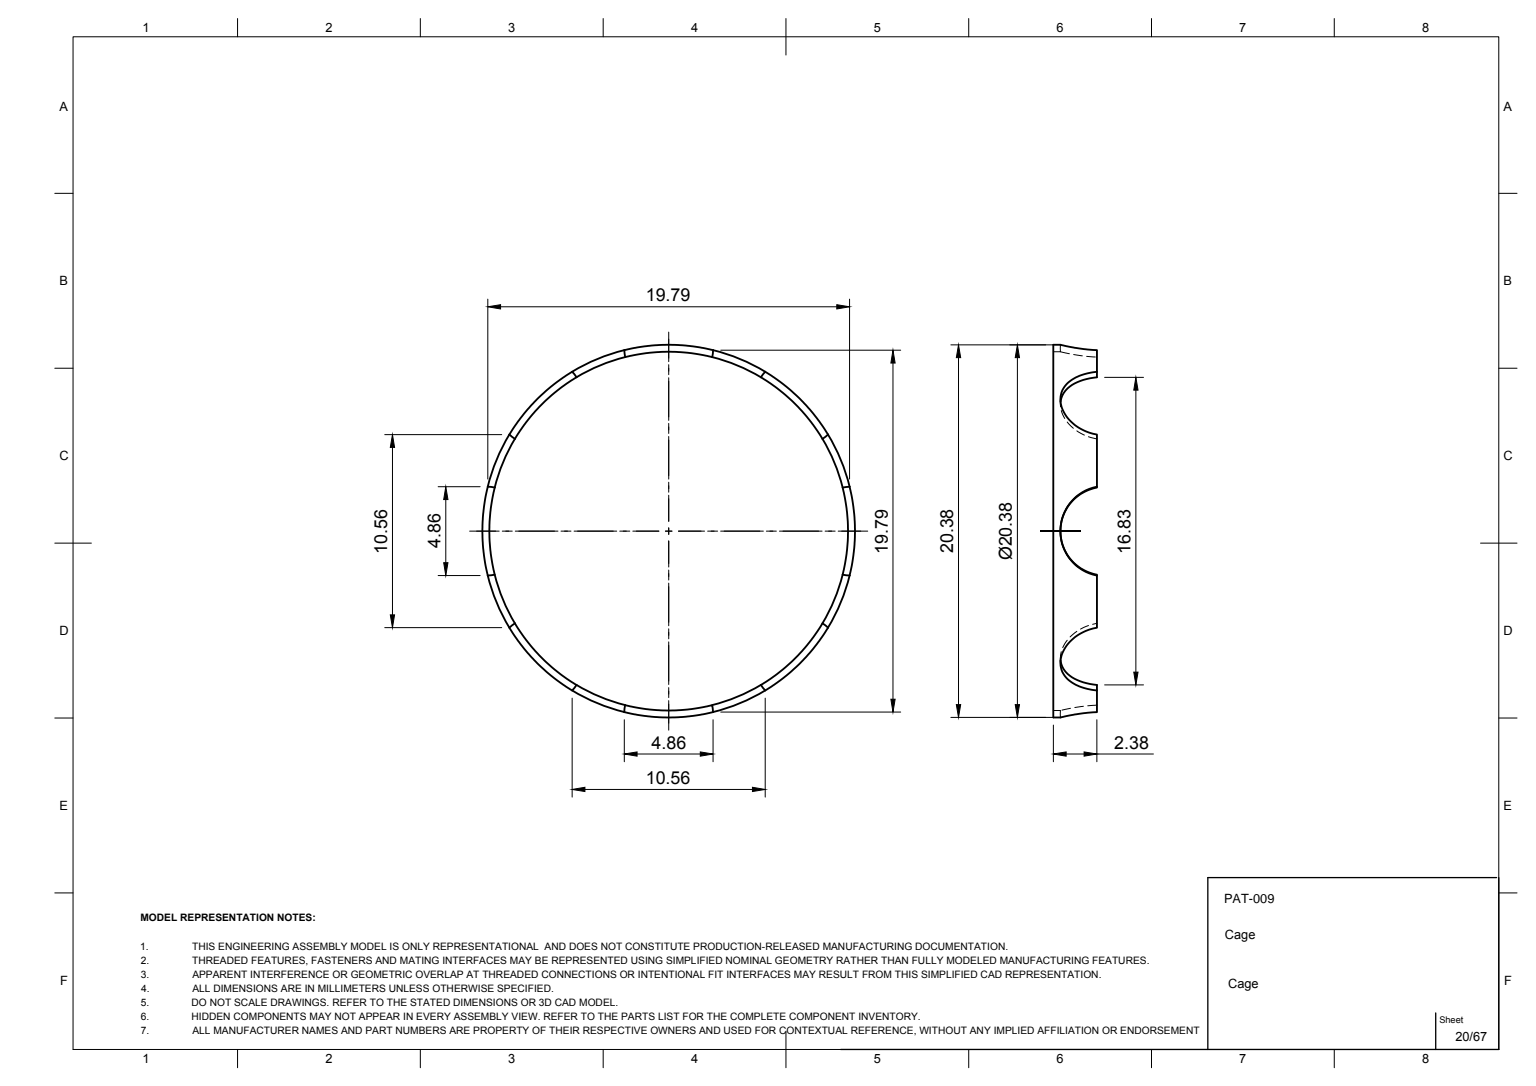
ISO-10303-21;
HEADER;
/* Generated by software containing ST-Developer
 * from STEP Tools, Inc. (www.steptools.com) 
 */

FILE_DESCRIPTION(
/* description */ ('Bell-crank linkage with push rods'),
/* implementation_level */ '2;1');

FILE_NAME(
/* name */ 'Cage.step',
/* time_stamp */ '2026-10-28T03:25:15-07:00',
/* author */ (''),
/* organization */ (''),
/* preprocessor_version */ 'ST-DEVELOPER v20.2',
/* originating_system */ 'Autodesk Translation Framework v15.17.0.0',
/* authorisation */ '');

FILE_SCHEMA (('AUTOMOTIVE_DESIGN { 1 0 10303 214 3 1 1 }'));
ENDSEC;

DATA;
#10=MECHANICAL_DESIGN_GEOMETRIC_PRESENTATION_REPRESENTATION('',(#624),#16678);
#423=SPHERICAL_SURFACE('',#9847,0.247676);
#424=SPHERICAL_SURFACE('',#9863,0.247676);
#425=SPHERICAL_SURFACE('',#9868,0.247676);
#426=SPHERICAL_SURFACE('',#9873,0.247676);
#427=SPHERICAL_SURFACE('',#9878,0.247676);
#428=SPHERICAL_SURFACE('',#9883,0.247676);
#429=SPHERICAL_SURFACE('',#9888,0.247676);
#430=SPHERICAL_SURFACE('',#9896,0.247676);
#473=B_SPLINE_CURVE_WITH_KNOTS('',3,(#14583,#14584,#14585,#14586,#14587,
#14588,#14589,#14590,#14591,#14592,#14593,#14594,#14595,#14596,#14597,#14598,
#14599,#14600,#14601,#14602,#14603,#14604),.UNSPECIFIED.,.F.,.F.,(4,2,2,
2,2,2,2,2,2,2,4),(0.0473477652366656,0.126350602536658,0.189525903804987,
0.252701205073317,0.313298422430275,0.373895639787233,0.434492857144191,
0.495090074501149,0.558265375769478,0.621440677037807,0.7004435143378),
 .UNSPECIFIED.);
#474=B_SPLINE_CURVE_WITH_KNOTS('',3,(#14608,#14609,#14610,#14611,#14612,
#14613,#14614,#14615,#14616,#14617,#14618,#14619,#14620,#14621,#14622,#14623,
#14624,#14625,#14626,#14627,#14628,#14629),.UNSPECIFIED.,.F.,.F.,(4,2,2,
2,2,2,2,2,2,2,4),(0.0464897534940957,0.0852567806515119,0.170513561303024,
0.246687263103517,0.308657850341199,0.370628437578881,0.432599024816563,
0.494569612054245,0.570743313854739,0.656000094506251,0.694767121663666),
 .UNSPECIFIED.);
#475=B_SPLINE_CURVE_WITH_KNOTS('',3,(#14635,#14636,#14637,#14638,#14639,
#14640,#14641,#14642,#14643,#14644,#14645,#14646,#14647,#14648,#14649,#14650,
#14651,#14652,#14653,#14654,#14655,#14656),.UNSPECIFIED.,.F.,.F.,(4,2,2,
2,2,2,2,2,2,2,4),(0.0464897534940957,0.0852567806515118,0.170513561303024,
0.246687263103517,0.308657850341199,0.370628437578881,0.432599024816563,
0.494569612054245,0.570743313854738,0.65600009450625,0.694767121663666),
 .UNSPECIFIED.);
#476=B_SPLINE_CURVE_WITH_KNOTS('',3,(#14660,#14661,#14662,#14663,#14664,
#14665,#14666,#14667,#14668,#14669,#14670,#14671,#14672,#14673,#14674,#14675,
#14676,#14677,#14678,#14679,#14680,#14681),.UNSPECIFIED.,.F.,.F.,(4,2,2,
2,2,2,2,2,2,2,4),(0.0464897534940957,0.0852567806515119,0.170513561303024,
0.246687263103517,0.308657850341199,0.370628437578881,0.432599024816563,
0.494569612054245,0.570743313854739,0.656000094506251,0.694767121663666),
 .UNSPECIFIED.);
#477=B_SPLINE_CURVE_WITH_KNOTS('',3,(#14685,#14686,#14687,#14688,#14689,
#14690,#14691,#14692,#14693,#14694,#14695,#14696),.UNSPECIFIED.,.F.,.F.,
(4,2,2,2,2,4),(0.0464897534940957,0.0852567806515119,0.170513561303024,
0.246687263103517,0.308657850341199,0.370628437578881),.UNSPECIFIED.);
#478=B_SPLINE_CURVE_WITH_KNOTS('',3,(#14701,#14702,#14703,#14704,#14705,
#14706,#14707,#14708,#14709,#14710,#14711,#14712),.UNSPECIFIED.,.F.,.F.,
(4,2,2,2,2,4),(0.370628437578881,0.432599024816563,0.494569612054245,0.570743313854738,
0.65600009450625,0.694767121663666),.UNSPECIFIED.);
#479=B_SPLINE_CURVE_WITH_KNOTS('',3,(#14716,#14717,#14718,#14719,#14720,
#14721,#14722,#14723,#14724,#14725,#14726,#14727,#14728,#14729,#14730,#14731,
#14732,#14733,#14734,#14735,#14736,#14737),.UNSPECIFIED.,.F.,.F.,(4,2,2,
2,2,2,2,2,2,2,4),(0.0464897534940957,0.0852567806515121,0.170513561303024,
0.246687263103518,0.308657850341199,0.370628437578881,0.432599024816563,
0.494569612054245,0.570743313854738,0.65600009450625,0.694767121663666),
 .UNSPECIFIED.);
#480=B_SPLINE_CURVE_WITH_KNOTS('',3,(#14741,#14742,#14743,#14744,#14745,
#14746,#14747,#14748,#14749,#14750,#14751,#14752,#14753,#14754,#14755,#14756,
#14757,#14758,#14759,#14760,#14761,#14762),.UNSPECIFIED.,.F.,.F.,(4,2,2,
2,2,2,2,2,2,2,4),(0.0464897534940957,0.0852567806515119,0.170513561303024,
0.246687263103517,0.308657850341199,0.370628437578881,0.432599024816563,
0.494569612054245,0.570743313854738,0.65600009450625,0.694767121663667),
 .UNSPECIFIED.);
#481=B_SPLINE_CURVE_WITH_KNOTS('',3,(#14766,#14767,#14768,#14769,#14770,
#14771,#14772,#14773,#14774,#14775,#14776,#14777,#14778,#14779,#14780,#14781,
#14782,#14783,#14784,#14785,#14786,#14787),.UNSPECIFIED.,.F.,.F.,(4,2,2,
2,2,2,2,2,2,2,4),(0.0464897534940957,0.0852567806515119,0.170513561303024,
0.246687263103517,0.308657850341199,0.370628437578881,0.432599024816563,
0.494569612054245,0.570743313854738,0.65600009450625,0.694767121663666),
 .UNSPECIFIED.);
#482=B_SPLINE_CURVE_WITH_KNOTS('',3,(#14791,#14792,#14793,#14794,#14795,
#14796,#14797,#14798,#14799,#14800,#14801,#14802,#14803,#14804,#14805,#14806,
#14807,#14808,#14809,#14810,#14811,#14812),.UNSPECIFIED.,.F.,.F.,(4,2,2,
2,2,2,2,2,2,2,4),(0.0464897534940957,0.0852567806515119,0.170513561303024,
0.246687263103517,0.308657850341199,0.370628437578881,0.432599024816563,
0.494569612054245,0.570743313854739,0.656000094506251,0.694767121663667),
 .UNSPECIFIED.);
#483=B_SPLINE_CURVE_WITH_KNOTS('',3,(#14820,#14821,#14822,#14823,#14824,
#14825,#14826,#14827,#14828,#14829,#14830,#14831,#14832,#14833,#14834,#14835,
#14836,#14837,#14838,#14839,#14840,#14841),.UNSPECIFIED.,.F.,.F.,(4,2,2,
2,2,2,2,2,2,2,4),(0.0473477652366656,0.126350602536658,0.189525903804987,
0.252701205073316,0.313298422430274,0.373895639787232,0.434492857144191,
0.495090074501149,0.558265375769478,0.621440677037807,0.7004435143378),
 .UNSPECIFIED.);
#484=B_SPLINE_CURVE_WITH_KNOTS('',3,(#14849,#14850,#14851,#14852,#14853,
#14854,#14855,#14856,#14857,#14858,#14859,#14860,#14861,#14862,#14863,#14864,
#14865,#14866,#14867,#14868,#14869,#14870),.UNSPECIFIED.,.F.,.F.,(4,2,2,
2,2,2,2,2,2,2,4),(0.0473477652366656,0.126350602536658,0.189525903804987,
0.252701205073317,0.313298422430275,0.373895639787233,0.434492857144191,
0.495090074501149,0.558265375769478,0.621440677037807,0.7004435143378),
 .UNSPECIFIED.);
#485=B_SPLINE_CURVE_WITH_KNOTS('',3,(#14879,#14880,#14881,#14882,#14883,
#14884,#14885,#14886,#14887,#14888,#14889,#14890),.UNSPECIFIED.,.F.,.F.,
(4,2,2,2,2,4),(0.0473477652366656,0.126350602536658,0.189525903804987,0.252701205073316,
0.313298422430275,0.373895639787233),.UNSPECIFIED.);
#486=B_SPLINE_CURVE_WITH_KNOTS('',3,(#14892,#14893,#14894,#14895,#14896,
#14897,#14898,#14899,#14900,#14901,#14902,#14903),.UNSPECIFIED.,.F.,.F.,
(4,2,2,2,2,4),(0.373895639787233,0.434492857144191,0.495090074501149,0.558265375769478,
0.621440677037807,0.7004435143378),.UNSPECIFIED.);
#487=B_SPLINE_CURVE_WITH_KNOTS('',3,(#14910,#14911,#14912,#14913,#14914,
#14915,#14916,#14917,#14918,#14919,#14920,#14921,#14922,#14923,#14924,#14925,
#14926,#14927,#14928,#14929,#14930,#14931),.UNSPECIFIED.,.F.,.F.,(4,2,2,
2,2,2,2,2,2,2,4),(0.0473477652366656,0.126350602536658,0.189525903804987,
0.252701205073316,0.313298422430275,0.373895639787233,0.434492857144191,
0.495090074501149,0.558265375769478,0.621440677037807,0.7004435143378),
 .UNSPECIFIED.);
#488=B_SPLINE_CURVE_WITH_KNOTS('',3,(#14939,#14940,#14941,#14942,#14943,
#14944,#14945,#14946,#14947,#14948,#14949,#14950,#14951,#14952,#14953,#14954,
#14955,#14956,#14957,#14958,#14959,#14960),.UNSPECIFIED.,.F.,.F.,(4,2,2,
2,2,2,2,2,2,2,4),(0.0473477652366656,0.126350602536658,0.189525903804987,
0.252701205073317,0.313298422430275,0.373895639787233,0.434492857144191,
0.495090074501149,0.558265375769478,0.621440677037807,0.7004435143378),
 .UNSPECIFIED.);
#489=B_SPLINE_CURVE_WITH_KNOTS('',3,(#14968,#14969,#14970,#14971,#14972,
#14973,#14974,#14975,#14976,#14977,#14978,#14979,#14980,#14981,#14982,#14983,
#14984,#14985,#14986,#14987,#14988,#14989),.UNSPECIFIED.,.F.,.F.,(4,2,2,
2,2,2,2,2,2,2,4),(0.0473477652366656,0.126350602536658,0.189525903804987,
0.252701205073316,0.313298422430275,0.373895639787233,0.434492857144191,
0.495090074501149,0.558265375769478,0.621440677037807,0.7004435143378),
 .UNSPECIFIED.);
#490=B_SPLINE_CURVE_WITH_KNOTS('',3,(#14998,#14999,#15000,#15001,#15002,
#15003,#15004,#15005,#15006,#15007,#15008,#15009,#15010,#15011,#15012,#15013,
#15014,#15015,#15016,#15017,#15018,#15019),.UNSPECIFIED.,.F.,.F.,(4,2,2,
2,2,2,2,2,2,2,4),(0.0473477652366656,0.126350602536658,0.189525903804987,
0.252701205073317,0.313298422430275,0.373895639787233,0.434492857144191,
0.495090074501149,0.558265375769478,0.621440677037807,0.7004435143378),
 .UNSPECIFIED.);
#509=SHAPE_REPRESENTATION_RELATIONSHIP('SRR','None',#16926,#563);
#563=ADVANCED_BREP_SHAPE_REPRESENTATION('',(#685),#16631);
#624=STYLED_ITEM('',(#17291),#685);
#685=MANIFOLD_SOLID_BREP('Continuous crown cage',#8815);
#817=FACE_BOUND('',#2066,.T.);
#1058=PLANE('',#9860);
#1059=PLANE('',#9865);
#1060=PLANE('',#9870);
#1061=PLANE('',#9875);
#1062=PLANE('',#9880);
#1063=PLANE('',#9885);
#1064=PLANE('',#9894);
#1065=PLANE('',#9898);
#1066=PLANE('',#9899);
#1434=FACE_OUTER_BOUND('',#2048,.T.);
#1435=FACE_OUTER_BOUND('',#2049,.T.);
#1436=FACE_OUTER_BOUND('',#2050,.T.);
#1437=FACE_OUTER_BOUND('',#2051,.T.);
#1438=FACE_OUTER_BOUND('',#2052,.T.);
#1439=FACE_OUTER_BOUND('',#2053,.T.);
#1440=FACE_OUTER_BOUND('',#2054,.T.);
#1441=FACE_OUTER_BOUND('',#2055,.T.);
#1442=FACE_OUTER_BOUND('',#2056,.T.);
#1443=FACE_OUTER_BOUND('',#2057,.T.);
#1444=FACE_OUTER_BOUND('',#2058,.T.);
#1445=FACE_OUTER_BOUND('',#2059,.T.);
#1446=FACE_OUTER_BOUND('',#2060,.T.);
#1447=FACE_OUTER_BOUND('',#2061,.T.);
#1448=FACE_OUTER_BOUND('',#2062,.T.);
#1449=FACE_OUTER_BOUND('',#2063,.T.);
#1450=FACE_OUTER_BOUND('',#2064,.T.);
#1451=FACE_OUTER_BOUND('',#2065,.T.);
#1452=FACE_OUTER_BOUND('',#2067,.T.);
#2048=EDGE_LOOP('',(#6755,#6756,#6757,#6758));
#2049=EDGE_LOOP('',(#6759,#6760,#6761,#6762,#6763,#6764,#6765,#6766,#6767,
#6768,#6769,#6770,#6771,#6772,#6773,#6774,#6775,#6776,#6777,#6778));
#2050=EDGE_LOOP('',(#6779,#6780,#6781,#6782));
#2051=EDGE_LOOP('',(#6783,#6784,#6785,#6786));
#2052=EDGE_LOOP('',(#6787,#6788,#6789,#6790));
#2053=EDGE_LOOP('',(#6791,#6792,#6793,#6794));
#2054=EDGE_LOOP('',(#6795,#6796,#6797,#6798));
#2055=EDGE_LOOP('',(#6799,#6800,#6801,#6802,#6803,#6804));
#2056=EDGE_LOOP('',(#6805,#6806,#6807,#6808));
#2057=EDGE_LOOP('',(#6809,#6810,#6811,#6812));
#2058=EDGE_LOOP('',(#6813,#6814,#6815,#6816));
#2059=EDGE_LOOP('',(#6817,#6818,#6819,#6820));
#2060=EDGE_LOOP('',(#6821,#6822,#6823,#6824));
#2061=EDGE_LOOP('',(#6825,#6826,#6827,#6828));
#2062=EDGE_LOOP('',(#6829,#6830,#6831,#6832,#6833,#6834,#6835,#6836,#6837,
#6838,#6839,#6840,#6841,#6842,#6843,#6844,#6845,#6846,#6847,#6848));
#2063=EDGE_LOOP('',(#6849,#6850,#6851,#6852));
#2064=EDGE_LOOP('',(#6853,#6854,#6855,#6856));
#2065=EDGE_LOOP('',(#6857));
#2066=EDGE_LOOP('',(#6858));
#2067=EDGE_LOOP('',(#6859,#6860,#6861,#6862));
#2749=LINE('',#14698,#3298);
#2750=LINE('',#14994,#3299);
#3298=VECTOR('',#11647,1.019052);
#3299=VECTOR('',#11724,0.980948);
#3819=CIRCLE('',#9848,0.243053047864041);
#3820=CIRCLE('',#9849,0.243053047864041);
#3821=CIRCLE('',#9851,1.019052);
#3822=CIRCLE('',#9852,1.019052);
#3823=CIRCLE('',#9853,1.019052);
#3824=CIRCLE('',#9854,1.019052);
#3825=CIRCLE('',#9855,1.019052);
#3826=CIRCLE('',#9856,1.019052);
#3827=CIRCLE('',#9857,1.019052);
#3828=CIRCLE('',#9858,1.019052);
#3829=CIRCLE('',#9859,1.019052);
#3830=CIRCLE('',#9861,0.980948);
#3831=CIRCLE('',#9862,0.243053047864041);
#3832=CIRCLE('',#9864,0.243053047864041);
#3833=CIRCLE('',#9866,0.980948);
#3834=CIRCLE('',#9867,0.243053047864041);
#3835=CIRCLE('',#9869,0.243053047864041);
#3836=CIRCLE('',#9871,0.980948);
#3837=CIRCLE('',#9872,0.243053047864041);
#3838=CIRCLE('',#9874,0.243053047864041);
#3839=CIRCLE('',#9876,0.980948);
#3840=CIRCLE('',#9877,0.243053047864041);
#3841=CIRCLE('',#9879,0.243053047864041);
#3842=CIRCLE('',#9881,0.980948);
#3843=CIRCLE('',#9882,0.243053047864041);
#3844=CIRCLE('',#9884,0.243053047864041);
#3845=CIRCLE('',#9886,0.980948);
#3846=CIRCLE('',#9887,0.243053047864041);
#3847=CIRCLE('',#9889,0.243053047864041);
#3848=CIRCLE('',#9891,0.980948);
#3849=CIRCLE('',#9892,0.980948);
#3850=CIRCLE('',#9893,0.980948);
#3851=CIRCLE('',#9895,0.243053047864041);
#3852=CIRCLE('',#9897,0.243053047864041);
#4399=VERTEX_POINT('',#14581);
#4400=VERTEX_POINT('',#14582);
#4401=VERTEX_POINT('',#14605);
#4402=VERTEX_POINT('',#14607);
#4403=VERTEX_POINT('',#14632);
#4404=VERTEX_POINT('',#14634);
#4405=VERTEX_POINT('',#14657);
#4406=VERTEX_POINT('',#14659);
#4407=VERTEX_POINT('',#14682);
#4408=VERTEX_POINT('',#14684);
#4409=VERTEX_POINT('',#14697);
#4410=VERTEX_POINT('',#14700);
#4411=VERTEX_POINT('',#14713);
#4412=VERTEX_POINT('',#14715);
#4413=VERTEX_POINT('',#14738);
#4414=VERTEX_POINT('',#14740);
#4415=VERTEX_POINT('',#14763);
#4416=VERTEX_POINT('',#14765);
#4417=VERTEX_POINT('',#14788);
#4418=VERTEX_POINT('',#14790);
#4419=VERTEX_POINT('',#14815);
#4420=VERTEX_POINT('',#14819);
#4421=VERTEX_POINT('',#14844);
#4422=VERTEX_POINT('',#14848);
#4423=VERTEX_POINT('',#14873);
#4424=VERTEX_POINT('',#14877);
#4425=VERTEX_POINT('',#14878);
#4426=VERTEX_POINT('',#14905);
#4427=VERTEX_POINT('',#14909);
#4428=VERTEX_POINT('',#14934);
#4429=VERTEX_POINT('',#14938);
#4430=VERTEX_POINT('',#14963);
#4431=VERTEX_POINT('',#14967);
#4432=VERTEX_POINT('',#14992);
#4433=VERTEX_POINT('',#14995);
#4434=VERTEX_POINT('',#14997);
#5255=EDGE_CURVE('',#4399,#4400,#473,.T.);
#5256=EDGE_CURVE('',#4401,#4399,#3819,.T.);
#5257=EDGE_CURVE('',#4402,#4401,#474,.T.);
#5258=EDGE_CURVE('',#4400,#4402,#3820,.T.);
#5259=EDGE_CURVE('',#4403,#4401,#3821,.T.);
#5260=EDGE_CURVE('',#4403,#4404,#475,.T.);
#5261=EDGE_CURVE('',#4405,#4404,#3822,.T.);
#5262=EDGE_CURVE('',#4405,#4406,#476,.T.);
#5263=EDGE_CURVE('',#4407,#4406,#3823,.T.);
#5264=EDGE_CURVE('',#4407,#4408,#477,.T.);
#5265=EDGE_CURVE('',#4408,#4409,#2749,.T.);
#5266=EDGE_CURVE('',#4409,#4409,#3824,.T.);
#5267=EDGE_CURVE('',#4408,#4410,#478,.T.);
#5268=EDGE_CURVE('',#4411,#4410,#3825,.T.);
#5269=EDGE_CURVE('',#4411,#4412,#479,.T.);
#5270=EDGE_CURVE('',#4413,#4412,#3826,.T.);
#5271=EDGE_CURVE('',#4413,#4414,#480,.T.);
#5272=EDGE_CURVE('',#4415,#4414,#3827,.T.);
#5273=EDGE_CURVE('',#4415,#4416,#481,.T.);
#5274=EDGE_CURVE('',#4417,#4416,#3828,.T.);
#5275=EDGE_CURVE('',#4417,#4418,#482,.T.);
#5276=EDGE_CURVE('',#4402,#4418,#3829,.T.);
#5277=EDGE_CURVE('',#4399,#4419,#3830,.T.);
#5278=EDGE_CURVE('',#4419,#4403,#3831,.T.);
#5279=EDGE_CURVE('',#4420,#4419,#483,.T.);
#5280=EDGE_CURVE('',#4404,#4420,#3832,.T.);
#5281=EDGE_CURVE('',#4420,#4421,#3833,.T.);
#5282=EDGE_CURVE('',#4421,#4405,#3834,.T.);
#5283=EDGE_CURVE('',#4422,#4421,#484,.T.);
#5284=EDGE_CURVE('',#4406,#4422,#3835,.T.);
#5285=EDGE_CURVE('',#4422,#4423,#3836,.T.);
#5286=EDGE_CURVE('',#4423,#4407,#3837,.T.);
#5287=EDGE_CURVE('',#4424,#4425,#485,.T.);
#5288=EDGE_CURVE('',#4410,#4424,#3838,.T.);
#5289=EDGE_CURVE('',#4425,#4423,#486,.T.);
#5290=EDGE_CURVE('',#4424,#4426,#3839,.T.);
#5291=EDGE_CURVE('',#4426,#4411,#3840,.T.);
#5292=EDGE_CURVE('',#4427,#4426,#487,.T.);
#5293=EDGE_CURVE('',#4412,#4427,#3841,.T.);
#5294=EDGE_CURVE('',#4427,#4428,#3842,.T.);
#5295=EDGE_CURVE('',#4428,#4413,#3843,.T.);
#5296=EDGE_CURVE('',#4429,#4428,#488,.T.);
#5297=EDGE_CURVE('',#4414,#4429,#3844,.T.);
#5298=EDGE_CURVE('',#4429,#4430,#3845,.T.);
#5299=EDGE_CURVE('',#4430,#4415,#3846,.T.);
#5300=EDGE_CURVE('',#4431,#4430,#489,.T.);
#5301=EDGE_CURVE('',#4416,#4431,#3847,.T.);
#5302=EDGE_CURVE('',#4432,#4432,#3848,.T.);
#5303=EDGE_CURVE('',#4432,#4425,#2750,.T.);
#5304=EDGE_CURVE('',#4433,#4400,#3849,.T.);
#5305=EDGE_CURVE('',#4433,#4434,#490,.T.);
#5306=EDGE_CURVE('',#4431,#4434,#3850,.T.);
#5307=EDGE_CURVE('',#4418,#4433,#3851,.T.);
#5308=EDGE_CURVE('',#4434,#4417,#3852,.T.);
#6755=ORIENTED_EDGE('',*,*,#5255,.F.);
#6756=ORIENTED_EDGE('',*,*,#5256,.F.);
#6757=ORIENTED_EDGE('',*,*,#5257,.F.);
#6758=ORIENTED_EDGE('',*,*,#5258,.F.);
#6759=ORIENTED_EDGE('',*,*,#5257,.T.);
#6760=ORIENTED_EDGE('',*,*,#5259,.F.);
#6761=ORIENTED_EDGE('',*,*,#5260,.T.);
#6762=ORIENTED_EDGE('',*,*,#5261,.F.);
#6763=ORIENTED_EDGE('',*,*,#5262,.T.);
#6764=ORIENTED_EDGE('',*,*,#5263,.F.);
#6765=ORIENTED_EDGE('',*,*,#5264,.T.);
#6766=ORIENTED_EDGE('',*,*,#5265,.T.);
#6767=ORIENTED_EDGE('',*,*,#5266,.F.);
#6768=ORIENTED_EDGE('',*,*,#5265,.F.);
#6769=ORIENTED_EDGE('',*,*,#5267,.T.);
#6770=ORIENTED_EDGE('',*,*,#5268,.F.);
#6771=ORIENTED_EDGE('',*,*,#5269,.T.);
#6772=ORIENTED_EDGE('',*,*,#5270,.F.);
#6773=ORIENTED_EDGE('',*,*,#5271,.T.);
#6774=ORIENTED_EDGE('',*,*,#5272,.F.);
#6775=ORIENTED_EDGE('',*,*,#5273,.T.);
#6776=ORIENTED_EDGE('',*,*,#5274,.F.);
#6777=ORIENTED_EDGE('',*,*,#5275,.T.);
#6778=ORIENTED_EDGE('',*,*,#5276,.F.);
#6779=ORIENTED_EDGE('',*,*,#5256,.T.);
#6780=ORIENTED_EDGE('',*,*,#5277,.T.);
#6781=ORIENTED_EDGE('',*,*,#5278,.T.);
#6782=ORIENTED_EDGE('',*,*,#5259,.T.);
#6783=ORIENTED_EDGE('',*,*,#5279,.F.);
#6784=ORIENTED_EDGE('',*,*,#5280,.F.);
#6785=ORIENTED_EDGE('',*,*,#5260,.F.);
#6786=ORIENTED_EDGE('',*,*,#5278,.F.);
#6787=ORIENTED_EDGE('',*,*,#5280,.T.);
#6788=ORIENTED_EDGE('',*,*,#5281,.T.);
#6789=ORIENTED_EDGE('',*,*,#5282,.T.);
#6790=ORIENTED_EDGE('',*,*,#5261,.T.);
#6791=ORIENTED_EDGE('',*,*,#5283,.F.);
#6792=ORIENTED_EDGE('',*,*,#5284,.F.);
#6793=ORIENTED_EDGE('',*,*,#5262,.F.);
#6794=ORIENTED_EDGE('',*,*,#5282,.F.);
#6795=ORIENTED_EDGE('',*,*,#5284,.T.);
#6796=ORIENTED_EDGE('',*,*,#5285,.T.);
#6797=ORIENTED_EDGE('',*,*,#5286,.T.);
#6798=ORIENTED_EDGE('',*,*,#5263,.T.);
#6799=ORIENTED_EDGE('',*,*,#5287,.F.);
#6800=ORIENTED_EDGE('',*,*,#5288,.F.);
#6801=ORIENTED_EDGE('',*,*,#5267,.F.);
#6802=ORIENTED_EDGE('',*,*,#5264,.F.);
#6803=ORIENTED_EDGE('',*,*,#5286,.F.);
#6804=ORIENTED_EDGE('',*,*,#5289,.F.);
#6805=ORIENTED_EDGE('',*,*,#5288,.T.);
#6806=ORIENTED_EDGE('',*,*,#5290,.T.);
#6807=ORIENTED_EDGE('',*,*,#5291,.T.);
#6808=ORIENTED_EDGE('',*,*,#5268,.T.);
#6809=ORIENTED_EDGE('',*,*,#5292,.F.);
#6810=ORIENTED_EDGE('',*,*,#5293,.F.);
#6811=ORIENTED_EDGE('',*,*,#5269,.F.);
#6812=ORIENTED_EDGE('',*,*,#5291,.F.);
#6813=ORIENTED_EDGE('',*,*,#5293,.T.);
#6814=ORIENTED_EDGE('',*,*,#5294,.T.);
#6815=ORIENTED_EDGE('',*,*,#5295,.T.);
#6816=ORIENTED_EDGE('',*,*,#5270,.T.);
#6817=ORIENTED_EDGE('',*,*,#5296,.F.);
#6818=ORIENTED_EDGE('',*,*,#5297,.F.);
#6819=ORIENTED_EDGE('',*,*,#5271,.F.);
#6820=ORIENTED_EDGE('',*,*,#5295,.F.);
#6821=ORIENTED_EDGE('',*,*,#5297,.T.);
#6822=ORIENTED_EDGE('',*,*,#5298,.T.);
#6823=ORIENTED_EDGE('',*,*,#5299,.T.);
#6824=ORIENTED_EDGE('',*,*,#5272,.T.);
#6825=ORIENTED_EDGE('',*,*,#5273,.F.);
#6826=ORIENTED_EDGE('',*,*,#5299,.F.);
#6827=ORIENTED_EDGE('',*,*,#5300,.F.);
#6828=ORIENTED_EDGE('',*,*,#5301,.F.);
#6829=ORIENTED_EDGE('',*,*,#5302,.F.);
#6830=ORIENTED_EDGE('',*,*,#5303,.T.);
#6831=ORIENTED_EDGE('',*,*,#5289,.T.);
#6832=ORIENTED_EDGE('',*,*,#5285,.F.);
#6833=ORIENTED_EDGE('',*,*,#5283,.T.);
#6834=ORIENTED_EDGE('',*,*,#5281,.F.);
#6835=ORIENTED_EDGE('',*,*,#5279,.T.);
#6836=ORIENTED_EDGE('',*,*,#5277,.F.);
#6837=ORIENTED_EDGE('',*,*,#5255,.T.);
#6838=ORIENTED_EDGE('',*,*,#5304,.F.);
#6839=ORIENTED_EDGE('',*,*,#5305,.T.);
#6840=ORIENTED_EDGE('',*,*,#5306,.F.);
#6841=ORIENTED_EDGE('',*,*,#5300,.T.);
#6842=ORIENTED_EDGE('',*,*,#5298,.F.);
#6843=ORIENTED_EDGE('',*,*,#5296,.T.);
#6844=ORIENTED_EDGE('',*,*,#5294,.F.);
#6845=ORIENTED_EDGE('',*,*,#5292,.T.);
#6846=ORIENTED_EDGE('',*,*,#5290,.F.);
#6847=ORIENTED_EDGE('',*,*,#5287,.T.);
#6848=ORIENTED_EDGE('',*,*,#5303,.F.);
#6849=ORIENTED_EDGE('',*,*,#5258,.T.);
#6850=ORIENTED_EDGE('',*,*,#5276,.T.);
#6851=ORIENTED_EDGE('',*,*,#5307,.T.);
#6852=ORIENTED_EDGE('',*,*,#5304,.T.);
#6853=ORIENTED_EDGE('',*,*,#5275,.F.);
#6854=ORIENTED_EDGE('',*,*,#5308,.F.);
#6855=ORIENTED_EDGE('',*,*,#5305,.F.);
#6856=ORIENTED_EDGE('',*,*,#5307,.F.);
#6857=ORIENTED_EDGE('',*,*,#5266,.T.);
#6858=ORIENTED_EDGE('',*,*,#5302,.T.);
#6859=ORIENTED_EDGE('',*,*,#5301,.T.);
#6860=ORIENTED_EDGE('',*,*,#5306,.T.);
#6861=ORIENTED_EDGE('',*,*,#5308,.T.);
#6862=ORIENTED_EDGE('',*,*,#5274,.T.);
#8145=CYLINDRICAL_SURFACE('',#9850,1.019052);
#8146=CYLINDRICAL_SURFACE('',#9890,0.980948);
#8459=ADVANCED_FACE('',(#1434),#423,.F.);
#8460=ADVANCED_FACE('',(#1435),#8145,.T.);
#8461=ADVANCED_FACE('',(#1436),#1058,.T.);
#8462=ADVANCED_FACE('',(#1437),#424,.F.);
#8463=ADVANCED_FACE('',(#1438),#1059,.T.);
#8464=ADVANCED_FACE('',(#1439),#425,.F.);
#8465=ADVANCED_FACE('',(#1440),#1060,.T.);
#8466=ADVANCED_FACE('',(#1441),#426,.F.);
#8467=ADVANCED_FACE('',(#1442),#1061,.T.);
#8468=ADVANCED_FACE('',(#1443),#427,.F.);
#8469=ADVANCED_FACE('',(#1444),#1062,.T.);
#8470=ADVANCED_FACE('',(#1445),#428,.F.);
#8471=ADVANCED_FACE('',(#1446),#1063,.T.);
#8472=ADVANCED_FACE('',(#1447),#429,.F.);
#8473=ADVANCED_FACE('',(#1448),#8146,.F.);
#8474=ADVANCED_FACE('',(#1449),#1064,.T.);
#8475=ADVANCED_FACE('',(#1450),#430,.F.);
#8476=ADVANCED_FACE('',(#1451,#817),#1065,.T.);
#8477=ADVANCED_FACE('',(#1452),#1066,.T.);
#8815=CLOSED_SHELL('',(#8459,#8460,#8461,#8462,#8463,#8464,#8465,#8466,
#8467,#8468,#8469,#8470,#8471,#8472,#8473,#8474,#8475,#8476,#8477));
#9846=AXIS2_PLACEMENT_3D('',#14579,#11631,#11632);
#9847=AXIS2_PLACEMENT_3D('',#14580,#11633,#11634);
#9848=AXIS2_PLACEMENT_3D('',#14606,#11635,#11636);
#9849=AXIS2_PLACEMENT_3D('',#14630,#11637,#11638);
#9850=AXIS2_PLACEMENT_3D('',#14631,#11639,#11640);
#9851=AXIS2_PLACEMENT_3D('',#14633,#11641,#11642);
#9852=AXIS2_PLACEMENT_3D('',#14658,#11643,#11644);
#9853=AXIS2_PLACEMENT_3D('',#14683,#11645,#11646);
#9854=AXIS2_PLACEMENT_3D('',#14699,#11648,#11649);
#9855=AXIS2_PLACEMENT_3D('',#14714,#11650,#11651);
#9856=AXIS2_PLACEMENT_3D('',#14739,#11652,#11653);
#9857=AXIS2_PLACEMENT_3D('',#14764,#11654,#11655);
#9858=AXIS2_PLACEMENT_3D('',#14789,#11656,#11657);
#9859=AXIS2_PLACEMENT_3D('',#14813,#11658,#11659);
#9860=AXIS2_PLACEMENT_3D('',#14814,#11660,#11661);
#9861=AXIS2_PLACEMENT_3D('',#14816,#11662,#11663);
#9862=AXIS2_PLACEMENT_3D('',#14817,#11664,#11665);
#9863=AXIS2_PLACEMENT_3D('',#14818,#11666,#11667);
#9864=AXIS2_PLACEMENT_3D('',#14842,#11668,#11669);
#9865=AXIS2_PLACEMENT_3D('',#14843,#11670,#11671);
#9866=AXIS2_PLACEMENT_3D('',#14845,#11672,#11673);
#9867=AXIS2_PLACEMENT_3D('',#14846,#11674,#11675);
#9868=AXIS2_PLACEMENT_3D('',#14847,#11676,#11677);
#9869=AXIS2_PLACEMENT_3D('',#14871,#11678,#11679);
#9870=AXIS2_PLACEMENT_3D('',#14872,#11680,#11681);
#9871=AXIS2_PLACEMENT_3D('',#14874,#11682,#11683);
#9872=AXIS2_PLACEMENT_3D('',#14875,#11684,#11685);
#9873=AXIS2_PLACEMENT_3D('',#14876,#11686,#11687);
#9874=AXIS2_PLACEMENT_3D('',#14891,#11688,#11689);
#9875=AXIS2_PLACEMENT_3D('',#14904,#11690,#11691);
#9876=AXIS2_PLACEMENT_3D('',#14906,#11692,#11693);
#9877=AXIS2_PLACEMENT_3D('',#14907,#11694,#11695);
#9878=AXIS2_PLACEMENT_3D('',#14908,#11696,#11697);
#9879=AXIS2_PLACEMENT_3D('',#14932,#11698,#11699);
#9880=AXIS2_PLACEMENT_3D('',#14933,#11700,#11701);
#9881=AXIS2_PLACEMENT_3D('',#14935,#11702,#11703);
#9882=AXIS2_PLACEMENT_3D('',#14936,#11704,#11705);
#9883=AXIS2_PLACEMENT_3D('',#14937,#11706,#11707);
#9884=AXIS2_PLACEMENT_3D('',#14961,#11708,#11709);
#9885=AXIS2_PLACEMENT_3D('',#14962,#11710,#11711);
#9886=AXIS2_PLACEMENT_3D('',#14964,#11712,#11713);
#9887=AXIS2_PLACEMENT_3D('',#14965,#11714,#11715);
#9888=AXIS2_PLACEMENT_3D('',#14966,#11716,#11717);
#9889=AXIS2_PLACEMENT_3D('',#14990,#11718,#11719);
#9890=AXIS2_PLACEMENT_3D('',#14991,#11720,#11721);
#9891=AXIS2_PLACEMENT_3D('',#14993,#11722,#11723);
#9892=AXIS2_PLACEMENT_3D('',#14996,#11725,#11726);
#9893=AXIS2_PLACEMENT_3D('',#15020,#11727,#11728);
#9894=AXIS2_PLACEMENT_3D('',#15021,#11729,#11730);
#9895=AXIS2_PLACEMENT_3D('',#15022,#11731,#11732);
#9896=AXIS2_PLACEMENT_3D('',#15023,#11733,#11734);
#9897=AXIS2_PLACEMENT_3D('',#15024,#11735,#11736);
#9898=AXIS2_PLACEMENT_3D('',#15025,#11737,#11738);
#9899=AXIS2_PLACEMENT_3D('',#15026,#11739,#11740);
#11631=DIRECTION('axis',(0.,0.,1.));
#11632=DIRECTION('refdir',(1.,0.,0.));
#11633=DIRECTION('center_axis',(0.,0.,1.));
#11634=DIRECTION('ref_axis',(1.,0.,0.));
#11635=DIRECTION('center_axis',(0.,-1.,0.));
#11636=DIRECTION('ref_axis',(0.,0.,-1.));
#11637=DIRECTION('center_axis',(0.,-1.,0.));
#11638=DIRECTION('ref_axis',(0.,0.,-1.));
#11639=DIRECTION('center_axis',(0.,1.,0.));
#11640=DIRECTION('ref_axis',(1.,0.,0.));
#11641=DIRECTION('center_axis',(0.,1.,0.));
#11642=DIRECTION('ref_axis',(1.,0.,0.));
#11643=DIRECTION('center_axis',(0.,1.,0.));
#11644=DIRECTION('ref_axis',(1.,0.,0.));
#11645=DIRECTION('center_axis',(0.,1.,0.));
#11646=DIRECTION('ref_axis',(1.,0.,0.));
#11647=DIRECTION('',(0.,-1.,0.));
#11648=DIRECTION('center_axis',(0.,-1.,0.));
#11649=DIRECTION('ref_axis',(1.,0.,0.));
#11650=DIRECTION('center_axis',(0.,1.,0.));
#11651=DIRECTION('ref_axis',(1.,0.,0.));
#11652=DIRECTION('center_axis',(0.,1.,0.));
#11653=DIRECTION('ref_axis',(1.,0.,0.));
#11654=DIRECTION('center_axis',(0.,1.,0.));
#11655=DIRECTION('ref_axis',(1.,0.,0.));
#11656=DIRECTION('center_axis',(0.,1.,0.));
#11657=DIRECTION('ref_axis',(1.,0.,0.));
#11658=DIRECTION('center_axis',(0.,1.,0.));
#11659=DIRECTION('ref_axis',(1.,0.,0.));
#11660=DIRECTION('center_axis',(0.,1.,0.));
#11661=DIRECTION('ref_axis',(1.,0.,0.));
#11662=DIRECTION('center_axis',(0.,-1.,0.));
#11663=DIRECTION('ref_axis',(1.,0.,0.));
#11664=DIRECTION('center_axis',(0.,-1.,0.));
#11665=DIRECTION('ref_axis',(0.,0.,-1.));
#11666=DIRECTION('center_axis',(6.12323399573677E-17,0.,1.));
#11667=DIRECTION('ref_axis',(1.,0.,0.));
#11668=DIRECTION('center_axis',(0.,-1.,0.));
#11669=DIRECTION('ref_axis',(0.,0.,-1.));
#11670=DIRECTION('center_axis',(0.,1.,0.));
#11671=DIRECTION('ref_axis',(1.,0.,0.));
#11672=DIRECTION('center_axis',(0.,-1.,0.));
#11673=DIRECTION('ref_axis',(1.,0.,0.));
#11674=DIRECTION('center_axis',(0.,-1.,0.));
#11675=DIRECTION('ref_axis',(0.,0.,-1.));
#11676=DIRECTION('center_axis',(0.,0.,1.));
#11677=DIRECTION('ref_axis',(1.,0.,0.));
#11678=DIRECTION('center_axis',(0.,-1.,0.));
#11679=DIRECTION('ref_axis',(0.,0.,-1.));
#11680=DIRECTION('center_axis',(0.,1.,0.));
#11681=DIRECTION('ref_axis',(1.,0.,0.));
#11682=DIRECTION('center_axis',(0.,-1.,0.));
#11683=DIRECTION('ref_axis',(1.,0.,0.));
#11684=DIRECTION('center_axis',(0.,-1.,0.));
#11685=DIRECTION('ref_axis',(0.,0.,-1.));
#11686=DIRECTION('center_axis',(0.,0.,1.));
#11687=DIRECTION('ref_axis',(1.,0.,0.));
#11688=DIRECTION('center_axis',(0.,-1.,0.));
#11689=DIRECTION('ref_axis',(0.,0.,-1.));
#11690=DIRECTION('center_axis',(0.,1.,0.));
#11691=DIRECTION('ref_axis',(1.,0.,0.));
#11692=DIRECTION('center_axis',(0.,-1.,0.));
#11693=DIRECTION('ref_axis',(1.,0.,0.));
#11694=DIRECTION('center_axis',(0.,-1.,0.));
#11695=DIRECTION('ref_axis',(0.,0.,-1.));
#11696=DIRECTION('center_axis',(0.,0.,1.));
#11697=DIRECTION('ref_axis',(1.,0.,0.));
#11698=DIRECTION('center_axis',(0.,-1.,0.));
#11699=DIRECTION('ref_axis',(0.,0.,-1.));
#11700=DIRECTION('center_axis',(0.,1.,0.));
#11701=DIRECTION('ref_axis',(1.,0.,0.));
#11702=DIRECTION('center_axis',(0.,-1.,0.));
#11703=DIRECTION('ref_axis',(1.,0.,0.));
#11704=DIRECTION('center_axis',(0.,-1.,0.));
#11705=DIRECTION('ref_axis',(0.,0.,-1.));
#11706=DIRECTION('center_axis',(6.12323399573676E-17,0.,1.));
#11707=DIRECTION('ref_axis',(1.,0.,0.));
#11708=DIRECTION('center_axis',(0.,-1.,0.));
#11709=DIRECTION('ref_axis',(0.,0.,-1.));
#11710=DIRECTION('center_axis',(0.,1.,0.));
#11711=DIRECTION('ref_axis',(1.,0.,0.));
#11712=DIRECTION('center_axis',(0.,-1.,0.));
#11713=DIRECTION('ref_axis',(1.,0.,0.));
#11714=DIRECTION('center_axis',(0.,-1.,0.));
#11715=DIRECTION('ref_axis',(0.,0.,-1.));
#11716=DIRECTION('center_axis',(0.,0.,1.));
#11717=DIRECTION('ref_axis',(1.,0.,0.));
#11718=DIRECTION('center_axis',(0.,-1.,0.));
#11719=DIRECTION('ref_axis',(0.,0.,-1.));
#11720=DIRECTION('center_axis',(0.,1.,0.));
#11721=DIRECTION('ref_axis',(1.,0.,0.));
#11722=DIRECTION('center_axis',(0.,1.,0.));
#11723=DIRECTION('ref_axis',(1.,0.,0.));
#11724=DIRECTION('',(0.,1.,0.));
#11725=DIRECTION('center_axis',(0.,-1.,0.));
#11726=DIRECTION('ref_axis',(1.,0.,0.));
#11727=DIRECTION('center_axis',(0.,-1.,0.));
#11728=DIRECTION('ref_axis',(1.,0.,0.));
#11729=DIRECTION('center_axis',(0.,1.,0.));
#11730=DIRECTION('ref_axis',(1.,0.,0.));
#11731=DIRECTION('center_axis',(0.,-1.,0.));
#11732=DIRECTION('ref_axis',(0.,0.,-1.));
#11733=DIRECTION('center_axis',(0.,0.,1.));
#11734=DIRECTION('ref_axis',(1.,0.,0.));
#11735=DIRECTION('center_axis',(0.,-1.,0.));
#11736=DIRECTION('ref_axis',(0.,0.,-1.));
#11737=DIRECTION('center_axis',(0.,-1.,0.));
#11738=DIRECTION('ref_axis',(-1.,0.,0.));
#11739=DIRECTION('center_axis',(0.,1.,0.));
#11740=DIRECTION('ref_axis',(1.,0.,0.));
#14579=CARTESIAN_POINT('',(0.,0.,0.));
#14580=CARTESIAN_POINT('Origin',(0.707106781186547,0.,0.707106781186548));
#14581=CARTESIAN_POINT('',(0.504455939115715,-0.04763,0.841298510752802));
#14582=CARTESIAN_POINT('',(0.841298510752802,-0.04763,0.504455939115715));
#14583=CARTESIAN_POINT('Ctrl Pts',(0.504455939115715,-0.04763,0.841298510752802));
#14584=CARTESIAN_POINT('Ctrl Pts',(0.508899795931835,-0.0740444353928835,
0.838633903678357));
#14585=CARTESIAN_POINT('Ctrl Pts',(0.517157748491652,-0.0999305678883309,
0.833661031856294));
#14586=CARTESIAN_POINT('Ctrl Pts',(0.537715343527944,-0.142345102874864,
0.820511285096538));
#14587=CARTESIAN_POINT('Ctrl Pts',(0.548874290046456,-0.159766064500479,
0.813159949759));
#14588=CARTESIAN_POINT('Ctrl Pts',(0.573915184558107,-0.190326085855194,
0.795684265985089));
#14589=CARTESIAN_POINT('Ctrl Pts',(0.587792702767295,-0.203463743702801,
0.78555112003688));
#14590=CARTESIAN_POINT('Ctrl Pts',(0.615966552324775,-0.224161999508995,
0.763642258217233));
#14591=CARTESIAN_POINT('Ctrl Pts',(0.631684198665438,-0.232861760990032,
0.750785745543687));
#14592=CARTESIAN_POINT('Ctrl Pts',(0.663382628119203,-0.244251601209411,
0.722929908501543));
#14593=CARTESIAN_POINT('Ctrl Pts',(0.679352081686668,-0.246942143572133,
0.707917883896095));
#14594=CARTESIAN_POINT('Ctrl Pts',(0.707917883896095,-0.246942143572133,
0.679352081686668));
#14595=CARTESIAN_POINT('Ctrl Pts',(0.722929908501543,-0.244251601209411,
0.663382628119203));
#14596=CARTESIAN_POINT('Ctrl Pts',(0.750785745543687,-0.232861760990032,
0.631684198665439));
#14597=CARTESIAN_POINT('Ctrl Pts',(0.763642258217232,-0.224161999508995,
0.615966552324775));
#14598=CARTESIAN_POINT('Ctrl Pts',(0.78555112003688,-0.203463743702801,
0.587792702767295));
#14599=CARTESIAN_POINT('Ctrl Pts',(0.795684265985088,-0.190326085855194,
0.573915184558108));
#14600=CARTESIAN_POINT('Ctrl Pts',(0.813159949759,-0.15976606450048,0.548874290046456));
#14601=CARTESIAN_POINT('Ctrl Pts',(0.820511285096538,-0.142345102874864,
0.537715343527944));
#14602=CARTESIAN_POINT('Ctrl Pts',(0.833661031856294,-0.099930567888331,
0.517157748491653));
#14603=CARTESIAN_POINT('Ctrl Pts',(0.838633903678357,-0.0740444353928835,
0.508899795931835));
#14604=CARTESIAN_POINT('Ctrl Pts',(0.841298510752801,-0.0476299999999999,
0.504455939115715));
#14605=CARTESIAN_POINT('',(0.528110872004958,-0.04763,0.871530771444223));
#14606=CARTESIAN_POINT('Origin',(0.707106781186547,-0.04763,0.707106781186548));
#14607=CARTESIAN_POINT('',(0.871530771444223,-0.04763,0.528110872004959));
#14608=CARTESIAN_POINT('Ctrl Pts',(0.871530771444223,-0.0476300000000001,
0.528110872004958));
#14609=CARTESIAN_POINT('Ctrl Pts',(0.87014664509073,-0.0609922781173483,
0.530395067942936));
#14610=CARTESIAN_POINT('Ctrl Pts',(0.868149331745851,-0.0742967091364493,
0.533674141594226));
#14611=CARTESIAN_POINT('Ctrl Pts',(0.85981294420286,-0.115492077056649,
0.54708917182331));
#14612=CARTESIAN_POINT('Ctrl Pts',(0.850993704737257,-0.141695629206859,
0.560922177770136));
#14613=CARTESIAN_POINT('Ctrl Pts',(0.830754510485543,-0.181890537957859,
0.590422647829571));
#14614=CARTESIAN_POINT('Ctrl Pts',(0.816896541396381,-0.201072148666545,
0.609616703125488));
#14615=CARTESIAN_POINT('Ctrl Pts',(0.792310597819928,-0.223955109275652,
0.641117951819998));
#14616=CARTESIAN_POINT('Ctrl Pts',(0.779109323683612,-0.232742381310829,
0.657208095763053));
#14617=CARTESIAN_POINT('Ctrl Pts',(0.750552691816206,-0.244234834628584,
0.68964083160521));
#14618=CARTESIAN_POINT('Ctrl Pts',(0.735185187071673,-0.246942143572133,
0.705971972091755));
#14619=CARTESIAN_POINT('Ctrl Pts',(0.705971972091754,-0.246942143572133,
0.735185187071673));
#14620=CARTESIAN_POINT('Ctrl Pts',(0.689640831605209,-0.244234834628584,
0.750552691816206));
#14621=CARTESIAN_POINT('Ctrl Pts',(0.657208095763052,-0.232742381310829,
0.779109323683612));
#14622=CARTESIAN_POINT('Ctrl Pts',(0.641117951819998,-0.223955109275652,
0.792310597819928));
#14623=CARTESIAN_POINT('Ctrl Pts',(0.609616703125487,-0.201072148666545,
0.816896541396382));
#14624=CARTESIAN_POINT('Ctrl Pts',(0.590422647829571,-0.181890537957858,
0.830754510485544));
#14625=CARTESIAN_POINT('Ctrl Pts',(0.560922177770135,-0.141695629206858,
0.850993704737257));
#14626=CARTESIAN_POINT('Ctrl Pts',(0.547089171823309,-0.115492077056649,
0.859812944202861));
#14627=CARTESIAN_POINT('Ctrl Pts',(0.533674141594226,-0.0742967091364491,
0.868149331745852));
#14628=CARTESIAN_POINT('Ctrl Pts',(0.530395067942936,-0.0609922781173483,
0.870146645090731));
#14629=CARTESIAN_POINT('Ctrl Pts',(0.528110872004958,-0.0476300000000001,
0.871530771444223));
#14630=CARTESIAN_POINT('Origin',(0.707106781186547,-0.04763,0.707106781186548));
#14631=CARTESIAN_POINT('Origin',(0.,-0.166705,0.));
#14632=CARTESIAN_POINT('',(0.242834539687906,-0.04763,0.989696097314));
#14633=CARTESIAN_POINT('Origin',(0.,-0.04763,0.));
#14634=CARTESIAN_POINT('',(-0.242834539687907,-0.04763,0.989696097314));
#14635=CARTESIAN_POINT('Ctrl Pts',(0.242834539687906,-0.04763,0.989696097314));
#14636=CARTESIAN_POINT('Ctrl Pts',(0.24024064412003,-0.0609922781173483,
0.990332542620729));
#14637=CARTESIAN_POINT('Ctrl Pts',(0.236509675094874,-0.0742967091364492,
0.991238884025248));
#14638=CARTESIAN_POINT('Ctrl Pts',(0.221129100087819,-0.115492077056649,
0.994830026707808));
#14639=CARTESIAN_POINT('Ctrl Pts',(0.205111543747588,-0.141695629206859,
0.998375294985966));
#14640=CARTESIAN_POINT('Ctrl Pts',(0.169940289819232,-0.181890537957859,
1.00492400591205));
#14641=CARTESIAN_POINT('Ctrl Pts',(0.1465689792446,-0.201072148666545,1.00869718865384));
#14642=CARTESIAN_POINT('Ctrl Pts',(0.106909345252087,-0.223955109275652,
1.01358704779679));
#14643=CARTESIAN_POINT('Ctrl Pts',(0.0861971848975941,-0.232742381310829,
1.0156297872271));
#14644=CARTESIAN_POINT('Ctrl Pts',(0.0430711894098822,-0.244234834628584,
1.01837060663223));
#14645=CARTESIAN_POINT('Ctrl Pts',(0.0206568624125605,-0.246942143572133,
1.019052));
#14646=CARTESIAN_POINT('Ctrl Pts',(-0.0206568624125608,-0.246942143572133,
1.019052));
#14647=CARTESIAN_POINT('Ctrl Pts',(-0.0430711894098825,-0.244234834628584,
1.01837060663223));
#14648=CARTESIAN_POINT('Ctrl Pts',(-0.0861971848975943,-0.232742381310829,
1.0156297872271));
#14649=CARTESIAN_POINT('Ctrl Pts',(-0.106909345252088,-0.223955109275652,
1.01358704779679));
#14650=CARTESIAN_POINT('Ctrl Pts',(-0.1465689792446,-0.201072148666545,
1.00869718865384));
#14651=CARTESIAN_POINT('Ctrl Pts',(-0.169940289819232,-0.181890537957859,
1.00492400591205));
#14652=CARTESIAN_POINT('Ctrl Pts',(-0.205111543747588,-0.141695629206859,
0.998375294985966));
#14653=CARTESIAN_POINT('Ctrl Pts',(-0.221129100087819,-0.115492077056649,
0.994830026707808));
#14654=CARTESIAN_POINT('Ctrl Pts',(-0.236509675094875,-0.0742967091364493,
0.991238884025248));
#14655=CARTESIAN_POINT('Ctrl Pts',(-0.24024064412003,-0.0609922781173483,
0.990332542620729));
#14656=CARTESIAN_POINT('Ctrl Pts',(-0.242834539687907,-0.04763,0.989696097314));
#14657=CARTESIAN_POINT('',(-0.528110872004959,-0.04763,0.871530771444223));
#14658=CARTESIAN_POINT('Origin',(0.,-0.04763,0.));
#14659=CARTESIAN_POINT('',(-0.871530771444223,-0.04763,0.528110872004958));
#14660=CARTESIAN_POINT('Ctrl Pts',(-0.528110872004958,-0.0476300000000001,
0.871530771444223));
#14661=CARTESIAN_POINT('Ctrl Pts',(-0.530395067942936,-0.0609922781173484,
0.87014664509073));
#14662=CARTESIAN_POINT('Ctrl Pts',(-0.533674141594226,-0.0742967091364493,
0.868149331745851));
#14663=CARTESIAN_POINT('Ctrl Pts',(-0.54708917182331,-0.115492077056649,
0.85981294420286));
#14664=CARTESIAN_POINT('Ctrl Pts',(-0.560922177770136,-0.141695629206859,
0.850993704737257));
#14665=CARTESIAN_POINT('Ctrl Pts',(-0.590422647829571,-0.181890537957859,
0.830754510485543));
#14666=CARTESIAN_POINT('Ctrl Pts',(-0.609616703125488,-0.201072148666545,
0.816896541396381));
#14667=CARTESIAN_POINT('Ctrl Pts',(-0.641117951819998,-0.223955109275652,
0.792310597819928));
#14668=CARTESIAN_POINT('Ctrl Pts',(-0.657208095763053,-0.232742381310829,
0.779109323683611));
#14669=CARTESIAN_POINT('Ctrl Pts',(-0.68964083160521,-0.244234834628584,
0.750552691816205));
#14670=CARTESIAN_POINT('Ctrl Pts',(-0.705971972091755,-0.246942143572133,
0.735185187071673));
#14671=CARTESIAN_POINT('Ctrl Pts',(-0.735185187071673,-0.246942143572133,
0.705971972091754));
#14672=CARTESIAN_POINT('Ctrl Pts',(-0.750552691816206,-0.244234834628584,
0.689640831605209));
#14673=CARTESIAN_POINT('Ctrl Pts',(-0.779109323683612,-0.232742381310829,
0.657208095763052));
#14674=CARTESIAN_POINT('Ctrl Pts',(-0.792310597819928,-0.223955109275652,
0.641117951819998));
#14675=CARTESIAN_POINT('Ctrl Pts',(-0.816896541396382,-0.201072148666545,
0.609616703125487));
#14676=CARTESIAN_POINT('Ctrl Pts',(-0.830754510485544,-0.181890537957858,
0.590422647829571));
#14677=CARTESIAN_POINT('Ctrl Pts',(-0.850993704737257,-0.141695629206858,
0.560922177770135));
#14678=CARTESIAN_POINT('Ctrl Pts',(-0.859812944202861,-0.115492077056649,
0.547089171823309));
#14679=CARTESIAN_POINT('Ctrl Pts',(-0.868149331745852,-0.0742967091364491,
0.533674141594226));
#14680=CARTESIAN_POINT('Ctrl Pts',(-0.870146645090731,-0.0609922781173483,
0.530395067942936));
#14681=CARTESIAN_POINT('Ctrl Pts',(-0.871530771444223,-0.04763,0.528110872004958));
#14682=CARTESIAN_POINT('',(-0.989696097314,-0.04763,0.242834539687906));
#14683=CARTESIAN_POINT('Origin',(0.,-0.04763,0.));
#14684=CARTESIAN_POINT('',(-1.019052,-0.246942143572133,1.248489836334E-16));
#14685=CARTESIAN_POINT('Ctrl Pts',(-0.989696097314,-0.04763,0.242834539687906));
#14686=CARTESIAN_POINT('Ctrl Pts',(-0.990332542620729,-0.0609922781173483,
0.24024064412003));
#14687=CARTESIAN_POINT('Ctrl Pts',(-0.991238884025248,-0.0742967091364492,
0.236509675094874));
#14688=CARTESIAN_POINT('Ctrl Pts',(-0.994830026707808,-0.115492077056649,
0.221129100087819));
#14689=CARTESIAN_POINT('Ctrl Pts',(-0.998375294985966,-0.141695629206859,
0.205111543747588));
#14690=CARTESIAN_POINT('Ctrl Pts',(-1.00492400591205,-0.181890537957859,
0.169940289819232));
#14691=CARTESIAN_POINT('Ctrl Pts',(-1.00869718865384,-0.201072148666545,
0.1465689792446));
#14692=CARTESIAN_POINT('Ctrl Pts',(-1.01358704779679,-0.223955109275652,
0.106909345252088));
#14693=CARTESIAN_POINT('Ctrl Pts',(-1.0156297872271,-0.232742381310829,
0.0861971848975944));
#14694=CARTESIAN_POINT('Ctrl Pts',(-1.01837060663223,-0.244234834628584,
0.0430711894098825));
#14695=CARTESIAN_POINT('Ctrl Pts',(-1.019052,-0.246942143572133,0.0206568624125608));
#14696=CARTESIAN_POINT('Ctrl Pts',(-1.019052,-0.246942143572133,1.2490009027033E-16));
#14697=CARTESIAN_POINT('',(-1.019052,-0.28578,1.24797876996471E-16));
#14698=CARTESIAN_POINT('',(-1.019052,-0.166705,1.24797876996471E-16));
#14699=CARTESIAN_POINT('Origin',(0.,-0.28578,0.));
#14700=CARTESIAN_POINT('',(-0.989696097314,-0.04763,-0.242834539687906));
#14701=CARTESIAN_POINT('Ctrl Pts',(-1.019052,-0.246942143572133,1.2490009027033E-16));
#14702=CARTESIAN_POINT('Ctrl Pts',(-1.019052,-0.246942143572133,-0.0206568624125605));
#14703=CARTESIAN_POINT('Ctrl Pts',(-1.01837060663223,-0.244234834628584,
-0.0430711894098822));
#14704=CARTESIAN_POINT('Ctrl Pts',(-1.0156297872271,-0.232742381310829,
-0.0861971848975941));
#14705=CARTESIAN_POINT('Ctrl Pts',(-1.01358704779679,-0.223955109275652,
-0.106909345252087));
#14706=CARTESIAN_POINT('Ctrl Pts',(-1.00869718865384,-0.201072148666546,
-0.1465689792446));
#14707=CARTESIAN_POINT('Ctrl Pts',(-1.00492400591205,-0.181890537957859,
-0.169940289819232));
#14708=CARTESIAN_POINT('Ctrl Pts',(-0.998375294985966,-0.141695629206859,
-0.205111543747588));
#14709=CARTESIAN_POINT('Ctrl Pts',(-0.994830026707808,-0.11549207705665,
-0.221129100087819));
#14710=CARTESIAN_POINT('Ctrl Pts',(-0.991238884025248,-0.0742967091364495,
-0.236509675094874));
#14711=CARTESIAN_POINT('Ctrl Pts',(-0.990332542620729,-0.0609922781173484,
-0.24024064412003));
#14712=CARTESIAN_POINT('Ctrl Pts',(-0.989696097314,-0.0476300000000001,
-0.242834539687907));
#14713=CARTESIAN_POINT('',(-0.871530771444223,-0.04763,-0.528110872004958));
#14714=CARTESIAN_POINT('Origin',(0.,-0.04763,0.));
#14715=CARTESIAN_POINT('',(-0.528110872004958,-0.04763,-0.871530771444223));
#14716=CARTESIAN_POINT('Ctrl Pts',(-0.871530771444223,-0.0476300000000001,
-0.528110872004958));
#14717=CARTESIAN_POINT('Ctrl Pts',(-0.87014664509073,-0.0609922781173484,
-0.530395067942936));
#14718=CARTESIAN_POINT('Ctrl Pts',(-0.868149331745851,-0.0742967091364494,
-0.533674141594226));
#14719=CARTESIAN_POINT('Ctrl Pts',(-0.85981294420286,-0.115492077056649,
-0.54708917182331));
#14720=CARTESIAN_POINT('Ctrl Pts',(-0.850993704737257,-0.141695629206859,
-0.560922177770136));
#14721=CARTESIAN_POINT('Ctrl Pts',(-0.830754510485543,-0.181890537957859,
-0.590422647829571));
#14722=CARTESIAN_POINT('Ctrl Pts',(-0.816896541396381,-0.201072148666546,
-0.609616703125488));
#14723=CARTESIAN_POINT('Ctrl Pts',(-0.792310597819928,-0.223955109275652,
-0.641117951819999));
#14724=CARTESIAN_POINT('Ctrl Pts',(-0.779109323683611,-0.232742381310829,
-0.657208095763053));
#14725=CARTESIAN_POINT('Ctrl Pts',(-0.750552691816205,-0.244234834628584,
-0.68964083160521));
#14726=CARTESIAN_POINT('Ctrl Pts',(-0.735185187071673,-0.246942143572133,
-0.705971972091755));
#14727=CARTESIAN_POINT('Ctrl Pts',(-0.705971972091754,-0.246942143572133,
-0.735185187071673));
#14728=CARTESIAN_POINT('Ctrl Pts',(-0.68964083160521,-0.244234834628584,
-0.750552691816206));
#14729=CARTESIAN_POINT('Ctrl Pts',(-0.657208095763052,-0.232742381310829,
-0.779109323683612));
#14730=CARTESIAN_POINT('Ctrl Pts',(-0.641117951819998,-0.223955109275652,
-0.792310597819928));
#14731=CARTESIAN_POINT('Ctrl Pts',(-0.609616703125488,-0.201072148666545,
-0.816896541396381));
#14732=CARTESIAN_POINT('Ctrl Pts',(-0.590422647829571,-0.181890537957859,
-0.830754510485543));
#14733=CARTESIAN_POINT('Ctrl Pts',(-0.560922177770136,-0.141695629206859,
-0.850993704737257));
#14734=CARTESIAN_POINT('Ctrl Pts',(-0.54708917182331,-0.115492077056649,
-0.85981294420286));
#14735=CARTESIAN_POINT('Ctrl Pts',(-0.533674141594226,-0.0742967091364494,
-0.868149331745852));
#14736=CARTESIAN_POINT('Ctrl Pts',(-0.530395067942936,-0.0609922781173484,
-0.870146645090731));
#14737=CARTESIAN_POINT('Ctrl Pts',(-0.528110872004958,-0.0476300000000001,
-0.871530771444223));
#14738=CARTESIAN_POINT('',(-0.242834539687906,-0.04763,-0.989696097314));
#14739=CARTESIAN_POINT('Origin',(0.,-0.04763,0.));
#14740=CARTESIAN_POINT('',(0.242834539687906,-0.04763,-0.989696097314));
#14741=CARTESIAN_POINT('Ctrl Pts',(-0.242834539687907,-0.04763,-0.989696097314));
#14742=CARTESIAN_POINT('Ctrl Pts',(-0.24024064412003,-0.0609922781173483,
-0.990332542620729));
#14743=CARTESIAN_POINT('Ctrl Pts',(-0.236509675094874,-0.0742967091364493,
-0.991238884025248));
#14744=CARTESIAN_POINT('Ctrl Pts',(-0.221129100087819,-0.115492077056649,
-0.994830026707808));
#14745=CARTESIAN_POINT('Ctrl Pts',(-0.205111543747588,-0.141695629206859,
-0.998375294985966));
#14746=CARTESIAN_POINT('Ctrl Pts',(-0.169940289819232,-0.181890537957859,
-1.00492400591205));
#14747=CARTESIAN_POINT('Ctrl Pts',(-0.1465689792446,-0.201072148666545,
-1.00869718865384));
#14748=CARTESIAN_POINT('Ctrl Pts',(-0.106909345252087,-0.223955109275652,
-1.01358704779679));
#14749=CARTESIAN_POINT('Ctrl Pts',(-0.0861971848975942,-0.232742381310829,
-1.0156297872271));
#14750=CARTESIAN_POINT('Ctrl Pts',(-0.0430711894098823,-0.244234834628584,
-1.01837060663223));
#14751=CARTESIAN_POINT('Ctrl Pts',(-0.0206568624125606,-0.246942143572133,
-1.019052));
#14752=CARTESIAN_POINT('Ctrl Pts',(0.0206568624125607,-0.246942143572133,
-1.019052));
#14753=CARTESIAN_POINT('Ctrl Pts',(0.0430711894098824,-0.244234834628584,
-1.01837060663223));
#14754=CARTESIAN_POINT('Ctrl Pts',(0.0861971848975943,-0.232742381310829,
-1.0156297872271));
#14755=CARTESIAN_POINT('Ctrl Pts',(0.106909345252088,-0.223955109275652,
-1.01358704779679));
#14756=CARTESIAN_POINT('Ctrl Pts',(0.1465689792446,-0.201072148666545,-1.00869718865384));
#14757=CARTESIAN_POINT('Ctrl Pts',(0.169940289819232,-0.181890537957859,
-1.00492400591205));
#14758=CARTESIAN_POINT('Ctrl Pts',(0.205111543747588,-0.141695629206859,
-0.998375294985966));
#14759=CARTESIAN_POINT('Ctrl Pts',(0.221129100087819,-0.115492077056649,
-0.994830026707808));
#14760=CARTESIAN_POINT('Ctrl Pts',(0.236509675094874,-0.0742967091364493,
-0.991238884025248));
#14761=CARTESIAN_POINT('Ctrl Pts',(0.24024064412003,-0.0609922781173484,
-0.990332542620729));
#14762=CARTESIAN_POINT('Ctrl Pts',(0.242834539687907,-0.04763,-0.989696097314));
#14763=CARTESIAN_POINT('',(0.528110872004958,-0.04763,-0.871530771444223));
#14764=CARTESIAN_POINT('Origin',(0.,-0.04763,0.));
#14765=CARTESIAN_POINT('',(0.871530771444223,-0.04763,-0.528110872004958));
#14766=CARTESIAN_POINT('Ctrl Pts',(0.528110872004958,-0.0476300000000001,
-0.871530771444223));
#14767=CARTESIAN_POINT('Ctrl Pts',(0.530395067942936,-0.0609922781173484,
-0.870146645090731));
#14768=CARTESIAN_POINT('Ctrl Pts',(0.533674141594226,-0.0742967091364493,
-0.868149331745851));
#14769=CARTESIAN_POINT('Ctrl Pts',(0.54708917182331,-0.115492077056649,
-0.85981294420286));
#14770=CARTESIAN_POINT('Ctrl Pts',(0.560922177770136,-0.141695629206859,
-0.850993704737257));
#14771=CARTESIAN_POINT('Ctrl Pts',(0.590422647829571,-0.181890537957859,
-0.830754510485543));
#14772=CARTESIAN_POINT('Ctrl Pts',(0.609616703125488,-0.201072148666545,
-0.816896541396381));
#14773=CARTESIAN_POINT('Ctrl Pts',(0.641117951819998,-0.223955109275652,
-0.792310597819928));
#14774=CARTESIAN_POINT('Ctrl Pts',(0.657208095763053,-0.232742381310829,
-0.779109323683612));
#14775=CARTESIAN_POINT('Ctrl Pts',(0.68964083160521,-0.244234834628584,
-0.750552691816206));
#14776=CARTESIAN_POINT('Ctrl Pts',(0.705971972091755,-0.246942143572133,
-0.735185187071673));
#14777=CARTESIAN_POINT('Ctrl Pts',(0.735185187071673,-0.246942143572133,
-0.705971972091754));
#14778=CARTESIAN_POINT('Ctrl Pts',(0.750552691816206,-0.244234834628584,
-0.68964083160521));
#14779=CARTESIAN_POINT('Ctrl Pts',(0.779109323683612,-0.232742381310829,
-0.657208095763053));
#14780=CARTESIAN_POINT('Ctrl Pts',(0.792310597819928,-0.223955109275652,
-0.641117951819998));
#14781=CARTESIAN_POINT('Ctrl Pts',(0.816896541396381,-0.201072148666545,
-0.609616703125488));
#14782=CARTESIAN_POINT('Ctrl Pts',(0.830754510485543,-0.181890537957859,
-0.590422647829571));
#14783=CARTESIAN_POINT('Ctrl Pts',(0.850993704737257,-0.141695629206859,
-0.560922177770136));
#14784=CARTESIAN_POINT('Ctrl Pts',(0.85981294420286,-0.115492077056649,
-0.54708917182331));
#14785=CARTESIAN_POINT('Ctrl Pts',(0.868149331745851,-0.0742967091364493,
-0.533674141594226));
#14786=CARTESIAN_POINT('Ctrl Pts',(0.870146645090731,-0.0609922781173484,
-0.530395067942936));
#14787=CARTESIAN_POINT('Ctrl Pts',(0.871530771444223,-0.0476300000000001,
-0.528110872004958));
#14788=CARTESIAN_POINT('',(0.989696097314,-0.04763,-0.242834539687906));
#14789=CARTESIAN_POINT('Origin',(0.,-0.04763,0.));
#14790=CARTESIAN_POINT('',(0.989696097314,-0.04763,0.242834539687906));
#14791=CARTESIAN_POINT('Ctrl Pts',(0.989696097314,-0.04763,-0.242834539687907));
#14792=CARTESIAN_POINT('Ctrl Pts',(0.990332542620729,-0.0609922781173483,
-0.24024064412003));
#14793=CARTESIAN_POINT('Ctrl Pts',(0.991238884025248,-0.0742967091364493,
-0.236509675094874));
#14794=CARTESIAN_POINT('Ctrl Pts',(0.994830026707808,-0.115492077056649,
-0.221129100087819));
#14795=CARTESIAN_POINT('Ctrl Pts',(0.998375294985966,-0.141695629206859,
-0.205111543747588));
#14796=CARTESIAN_POINT('Ctrl Pts',(1.00492400591205,-0.181890537957859,
-0.169940289819232));
#14797=CARTESIAN_POINT('Ctrl Pts',(1.00869718865384,-0.201072148666545,
-0.1465689792446));
#14798=CARTESIAN_POINT('Ctrl Pts',(1.01358704779679,-0.223955109275652,
-0.106909345252087));
#14799=CARTESIAN_POINT('Ctrl Pts',(1.0156297872271,-0.232742381310829,-0.0861971848975942));
#14800=CARTESIAN_POINT('Ctrl Pts',(1.01837060663223,-0.244234834628584,
-0.0430711894098823));
#14801=CARTESIAN_POINT('Ctrl Pts',(1.019052,-0.246942143572133,-0.0206568624125607));
#14802=CARTESIAN_POINT('Ctrl Pts',(1.019052,-0.246942143572133,0.0206568624125607));
#14803=CARTESIAN_POINT('Ctrl Pts',(1.01837060663223,-0.244234834628584,
0.0430711894098823));
#14804=CARTESIAN_POINT('Ctrl Pts',(1.0156297872271,-0.232742381310829,0.0861971848975942));
#14805=CARTESIAN_POINT('Ctrl Pts',(1.01358704779679,-0.223955109275652,
0.106909345252087));
#14806=CARTESIAN_POINT('Ctrl Pts',(1.00869718865384,-0.201072148666545,
0.1465689792446));
#14807=CARTESIAN_POINT('Ctrl Pts',(1.00492400591205,-0.181890537957859,
0.169940289819232));
#14808=CARTESIAN_POINT('Ctrl Pts',(0.998375294985966,-0.141695629206859,
0.205111543747588));
#14809=CARTESIAN_POINT('Ctrl Pts',(0.994830026707808,-0.115492077056649,
0.221129100087819));
#14810=CARTESIAN_POINT('Ctrl Pts',(0.991238884025248,-0.0742967091364492,
0.236509675094874));
#14811=CARTESIAN_POINT('Ctrl Pts',(0.990332542620729,-0.0609922781173483,
0.24024064412003));
#14812=CARTESIAN_POINT('Ctrl Pts',(0.989696097314,-0.04763,0.242834539687907));
#14813=CARTESIAN_POINT('Origin',(0.,-0.04763,0.));
#14814=CARTESIAN_POINT('Origin',(0.,-0.04763,0.));
#14815=CARTESIAN_POINT('',(0.238183666596899,-0.04763,0.951592097314));
#14816=CARTESIAN_POINT('Origin',(0.,-0.04763,0.));
#14817=CARTESIAN_POINT('Origin',(-1.94289029309402E-16,-0.04763,1.));
#14818=CARTESIAN_POINT('Origin',(-1.94289029309402E-16,0.,1.));
#14819=CARTESIAN_POINT('',(-0.2381836665969,-0.04763,0.951592097314));
#14820=CARTESIAN_POINT('Ctrl Pts',(-0.238183666596899,-0.0476299999999999,
0.951592097314));
#14821=CARTESIAN_POINT('Ctrl Pts',(-0.233157223576062,-0.0740444353928835,
0.952850216871763));
#14822=CARTESIAN_POINT('Ctrl Pts',(-0.223801617934946,-0.0999305678883309,
0.955173119738174));
#14823=CARTESIAN_POINT('Ctrl Pts',(-0.199966927975188,-0.142345102874864,
0.960411259488514));
#14824=CARTESIAN_POINT('Ctrl Pts',(-0.1868781821531,-0.159766064500479,
0.963103647174702));
#14825=CARTESIAN_POINT('Ctrl Pts',(-0.15681442133453,-0.190326085855194,
0.968453058988463));
#14826=CARTESIAN_POINT('Ctrl Pts',(-0.139836317888043,-0.203463743702801,
0.971100730005489));
#14827=CARTESIAN_POINT('Ctrl Pts',(-0.104422493053067,-0.224161999508995,
0.975530745318961));
#14828=CARTESIAN_POINT('Ctrl Pts',(-0.0842175114474176,-0.232861760990032,
0.977553872336861));
#14829=CARTESIAN_POINT('Ctrl Pts',(-0.0421062857595701,-0.244251601209411,
0.980270995488453));
#14830=CARTESIAN_POINT('Ctrl Pts',(-0.0201990724523197,-0.246942143572133,
0.980948));
#14831=CARTESIAN_POINT('Ctrl Pts',(0.020199072452319,-0.246942143572133,
0.980948));
#14832=CARTESIAN_POINT('Ctrl Pts',(0.0421062857595694,-0.244251601209411,
0.980270995488454));
#14833=CARTESIAN_POINT('Ctrl Pts',(0.0842175114474169,-0.232861760990032,
0.977553872336861));
#14834=CARTESIAN_POINT('Ctrl Pts',(0.104422493053067,-0.224161999508995,
0.975530745318961));
#14835=CARTESIAN_POINT('Ctrl Pts',(0.139836317888042,-0.203463743702801,
0.971100730005489));
#14836=CARTESIAN_POINT('Ctrl Pts',(0.15681442133453,-0.190326085855194,
0.968453058988463));
#14837=CARTESIAN_POINT('Ctrl Pts',(0.1868781821531,-0.15976606450048,0.963103647174702));
#14838=CARTESIAN_POINT('Ctrl Pts',(0.199966927975188,-0.142345102874864,
0.960411259488514));
#14839=CARTESIAN_POINT('Ctrl Pts',(0.223801617934945,-0.0999305678883309,
0.955173119738174));
#14840=CARTESIAN_POINT('Ctrl Pts',(0.233157223576061,-0.0740444353928835,
0.952850216871763));
#14841=CARTESIAN_POINT('Ctrl Pts',(0.238183666596899,-0.0476299999999999,
0.951592097314));
#14842=CARTESIAN_POINT('Origin',(-1.94289029309402E-16,-0.04763,1.));
#14843=CARTESIAN_POINT('Origin',(0.,-0.04763,0.));
#14844=CARTESIAN_POINT('',(-0.504455939115715,-0.04763,0.841298510752802));
#14845=CARTESIAN_POINT('Origin',(0.,-0.04763,0.));
#14846=CARTESIAN_POINT('Origin',(-0.707106781186548,-0.04763,0.707106781186547));
#14847=CARTESIAN_POINT('Origin',(-0.707106781186548,0.,0.707106781186547));
#14848=CARTESIAN_POINT('',(-0.841298510752802,-0.04763,0.504455939115715));
#14849=CARTESIAN_POINT('Ctrl Pts',(-0.841298510752802,-0.04763,0.504455939115715));
#14850=CARTESIAN_POINT('Ctrl Pts',(-0.838633903678357,-0.0740444353928835,
0.508899795931835));
#14851=CARTESIAN_POINT('Ctrl Pts',(-0.833661031856294,-0.0999305678883309,
0.517157748491652));
#14852=CARTESIAN_POINT('Ctrl Pts',(-0.820511285096538,-0.142345102874864,
0.537715343527944));
#14853=CARTESIAN_POINT('Ctrl Pts',(-0.813159949759,-0.159766064500479,0.548874290046456));
#14854=CARTESIAN_POINT('Ctrl Pts',(-0.795684265985089,-0.190326085855194,
0.573915184558107));
#14855=CARTESIAN_POINT('Ctrl Pts',(-0.78555112003688,-0.203463743702801,
0.587792702767295));
#14856=CARTESIAN_POINT('Ctrl Pts',(-0.763642258217233,-0.224161999508995,
0.615966552324775));
#14857=CARTESIAN_POINT('Ctrl Pts',(-0.750785745543687,-0.232861760990032,
0.631684198665438));
#14858=CARTESIAN_POINT('Ctrl Pts',(-0.722929908501543,-0.244251601209411,
0.663382628119203));
#14859=CARTESIAN_POINT('Ctrl Pts',(-0.707917883896095,-0.246942143572133,
0.679352081686668));
#14860=CARTESIAN_POINT('Ctrl Pts',(-0.679352081686668,-0.246942143572133,
0.707917883896095));
#14861=CARTESIAN_POINT('Ctrl Pts',(-0.663382628119203,-0.244251601209411,
0.722929908501544));
#14862=CARTESIAN_POINT('Ctrl Pts',(-0.631684198665438,-0.232861760990031,
0.750785745543687));
#14863=CARTESIAN_POINT('Ctrl Pts',(-0.615966552324775,-0.224161999508995,
0.763642258217233));
#14864=CARTESIAN_POINT('Ctrl Pts',(-0.587792702767295,-0.203463743702801,
0.78555112003688));
#14865=CARTESIAN_POINT('Ctrl Pts',(-0.573915184558107,-0.190326085855194,
0.795684265985088));
#14866=CARTESIAN_POINT('Ctrl Pts',(-0.548874290046456,-0.159766064500479,
0.813159949759));
#14867=CARTESIAN_POINT('Ctrl Pts',(-0.537715343527944,-0.142345102874864,
0.820511285096538));
#14868=CARTESIAN_POINT('Ctrl Pts',(-0.517157748491652,-0.0999305678883309,
0.833661031856294));
#14869=CARTESIAN_POINT('Ctrl Pts',(-0.508899795931835,-0.0740444353928835,
0.838633903678357));
#14870=CARTESIAN_POINT('Ctrl Pts',(-0.504455939115716,-0.04763,0.841298510752801));
#14871=CARTESIAN_POINT('Origin',(-0.707106781186548,-0.04763,0.707106781186547));
#14872=CARTESIAN_POINT('Origin',(0.,-0.04763,0.));
#14873=CARTESIAN_POINT('',(-0.951592097314,-0.04763,0.238183666596899));
#14874=CARTESIAN_POINT('Origin',(0.,-0.04763,0.));
#14875=CARTESIAN_POINT('Origin',(-1.,-0.04763,-1.11022302462516E-16));
#14876=CARTESIAN_POINT('Origin',(-1.,0.,-1.11022302462516E-16));
#14877=CARTESIAN_POINT('',(-0.951592097314,-0.04763,-0.2381836665969));
#14878=CARTESIAN_POINT('',(-0.980948,-0.246942143572133,1.08514323328844E-18));
#14879=CARTESIAN_POINT('Ctrl Pts',(-0.951592097314,-0.04763,-0.238183666596899));
#14880=CARTESIAN_POINT('Ctrl Pts',(-0.952850216871763,-0.0740444353928835,
-0.233157223576062));
#14881=CARTESIAN_POINT('Ctrl Pts',(-0.955173119738174,-0.0999305678883309,
-0.223801617934946));
#14882=CARTESIAN_POINT('Ctrl Pts',(-0.960411259488514,-0.142345102874864,
-0.199966927975188));
#14883=CARTESIAN_POINT('Ctrl Pts',(-0.963103647174702,-0.159766064500479,
-0.1868781821531));
#14884=CARTESIAN_POINT('Ctrl Pts',(-0.968453058988463,-0.190326085855194,
-0.15681442133453));
#14885=CARTESIAN_POINT('Ctrl Pts',(-0.971100730005489,-0.203463743702801,
-0.139836317888043));
#14886=CARTESIAN_POINT('Ctrl Pts',(-0.975530745318961,-0.224161999508995,
-0.104422493053067));
#14887=CARTESIAN_POINT('Ctrl Pts',(-0.977553872336861,-0.232861760990032,
-0.0842175114474175));
#14888=CARTESIAN_POINT('Ctrl Pts',(-0.980270995488453,-0.244251601209411,
-0.0421062857595699));
#14889=CARTESIAN_POINT('Ctrl Pts',(-0.980948,-0.246942143572133,-0.0201990724523195));
#14890=CARTESIAN_POINT('Ctrl Pts',(-0.980948,-0.246942143572133,-1.17961196366423E-16));
#14891=CARTESIAN_POINT('Origin',(-1.,-0.04763,-1.11022302462516E-16));
#14892=CARTESIAN_POINT('Ctrl Pts',(-0.980948,-0.246942143572133,-1.17961196366423E-16));
#14893=CARTESIAN_POINT('Ctrl Pts',(-0.980948,-0.246942143572133,0.0201990724523192));
#14894=CARTESIAN_POINT('Ctrl Pts',(-0.980270995488453,-0.244251601209411,
0.0421062857595695));
#14895=CARTESIAN_POINT('Ctrl Pts',(-0.977553872336861,-0.232861760990032,
0.0842175114474169));
#14896=CARTESIAN_POINT('Ctrl Pts',(-0.975530745318961,-0.224161999508995,
0.104422493053066));
#14897=CARTESIAN_POINT('Ctrl Pts',(-0.971100730005489,-0.203463743702801,
0.139836317888042));
#14898=CARTESIAN_POINT('Ctrl Pts',(-0.968453058988463,-0.190326085855194,
0.15681442133453));
#14899=CARTESIAN_POINT('Ctrl Pts',(-0.963103647174702,-0.15976606450048,
0.1868781821531));
#14900=CARTESIAN_POINT('Ctrl Pts',(-0.960411259488514,-0.142345102874864,
0.199966927975188));
#14901=CARTESIAN_POINT('Ctrl Pts',(-0.955173119738174,-0.099930567888331,
0.223801617934945));
#14902=CARTESIAN_POINT('Ctrl Pts',(-0.952850216871763,-0.0740444353928835,
0.233157223576061));
#14903=CARTESIAN_POINT('Ctrl Pts',(-0.951592097314,-0.04763,0.238183666596899));
#14904=CARTESIAN_POINT('Origin',(0.,-0.04763,0.));
#14905=CARTESIAN_POINT('',(-0.841298510752802,-0.04763,-0.504455939115715));
#14906=CARTESIAN_POINT('Origin',(0.,-0.04763,0.));
#14907=CARTESIAN_POINT('Origin',(-0.707106781186547,-0.04763,-0.707106781186548));
#14908=CARTESIAN_POINT('Origin',(-0.707106781186547,0.,-0.707106781186548));
#14909=CARTESIAN_POINT('',(-0.504455939115715,-0.04763,-0.841298510752802));
#14910=CARTESIAN_POINT('Ctrl Pts',(-0.504455939115715,-0.04763,-0.841298510752802));
#14911=CARTESIAN_POINT('Ctrl Pts',(-0.508899795931835,-0.0740444353928835,
-0.838633903678357));
#14912=CARTESIAN_POINT('Ctrl Pts',(-0.517157748491652,-0.0999305678883309,
-0.833661031856294));
#14913=CARTESIAN_POINT('Ctrl Pts',(-0.537715343527944,-0.142345102874864,
-0.820511285096538));
#14914=CARTESIAN_POINT('Ctrl Pts',(-0.548874290046456,-0.159766064500479,
-0.813159949759));
#14915=CARTESIAN_POINT('Ctrl Pts',(-0.573915184558107,-0.190326085855194,
-0.795684265985089));
#14916=CARTESIAN_POINT('Ctrl Pts',(-0.587792702767295,-0.203463743702801,
-0.78555112003688));
#14917=CARTESIAN_POINT('Ctrl Pts',(-0.615966552324775,-0.224161999508995,
-0.763642258217233));
#14918=CARTESIAN_POINT('Ctrl Pts',(-0.631684198665438,-0.232861760990032,
-0.750785745543687));
#14919=CARTESIAN_POINT('Ctrl Pts',(-0.663382628119203,-0.244251601209411,
-0.722929908501543));
#14920=CARTESIAN_POINT('Ctrl Pts',(-0.679352081686668,-0.246942143572133,
-0.707917883896095));
#14921=CARTESIAN_POINT('Ctrl Pts',(-0.707917883896095,-0.246942143572133,
-0.679352081686668));
#14922=CARTESIAN_POINT('Ctrl Pts',(-0.722929908501543,-0.244251601209411,
-0.663382628119203));
#14923=CARTESIAN_POINT('Ctrl Pts',(-0.750785745543687,-0.232861760990032,
-0.631684198665439));
#14924=CARTESIAN_POINT('Ctrl Pts',(-0.763642258217232,-0.224161999508995,
-0.615966552324775));
#14925=CARTESIAN_POINT('Ctrl Pts',(-0.78555112003688,-0.203463743702801,
-0.587792702767295));
#14926=CARTESIAN_POINT('Ctrl Pts',(-0.795684265985088,-0.190326085855194,
-0.573915184558107));
#14927=CARTESIAN_POINT('Ctrl Pts',(-0.813159949759,-0.15976606450048,-0.548874290046456));
#14928=CARTESIAN_POINT('Ctrl Pts',(-0.820511285096538,-0.142345102874864,
-0.537715343527944));
#14929=CARTESIAN_POINT('Ctrl Pts',(-0.833661031856294,-0.0999305678883311,
-0.517157748491652));
#14930=CARTESIAN_POINT('Ctrl Pts',(-0.838633903678357,-0.0740444353928836,
-0.508899795931835));
#14931=CARTESIAN_POINT('Ctrl Pts',(-0.841298510752801,-0.04763,-0.504455939115715));
#14932=CARTESIAN_POINT('Origin',(-0.707106781186547,-0.04763,-0.707106781186548));
#14933=CARTESIAN_POINT('Origin',(0.,-0.04763,0.));
#14934=CARTESIAN_POINT('',(-0.238183666596899,-0.04763,-0.951592097314));
#14935=CARTESIAN_POINT('Origin',(0.,-0.04763,0.));
#14936=CARTESIAN_POINT('Origin',(5.55111512312578E-17,-0.04763,-1.));
#14937=CARTESIAN_POINT('Origin',(5.55111512312578E-17,0.,-1.));
#14938=CARTESIAN_POINT('',(0.238183666596899,-0.04763,-0.951592097314));
#14939=CARTESIAN_POINT('Ctrl Pts',(0.238183666596899,-0.04763,-0.951592097314));
#14940=CARTESIAN_POINT('Ctrl Pts',(0.233157223576062,-0.0740444353928835,
-0.952850216871763));
#14941=CARTESIAN_POINT('Ctrl Pts',(0.223801617934946,-0.099930567888331,
-0.955173119738174));
#14942=CARTESIAN_POINT('Ctrl Pts',(0.199966927975188,-0.142345102874864,
-0.960411259488514));
#14943=CARTESIAN_POINT('Ctrl Pts',(0.1868781821531,-0.15976606450048,-0.963103647174702));
#14944=CARTESIAN_POINT('Ctrl Pts',(0.15681442133453,-0.190326085855194,
-0.968453058988463));
#14945=CARTESIAN_POINT('Ctrl Pts',(0.139836317888042,-0.203463743702801,
-0.971100730005489));
#14946=CARTESIAN_POINT('Ctrl Pts',(0.104422493053067,-0.224161999508995,
-0.975530745318961));
#14947=CARTESIAN_POINT('Ctrl Pts',(0.0842175114474173,-0.232861760990032,
-0.977553872336861));
#14948=CARTESIAN_POINT('Ctrl Pts',(0.0421062857595698,-0.244251601209411,
-0.980270995488453));
#14949=CARTESIAN_POINT('Ctrl Pts',(0.0201990724523194,-0.246942143572133,
-0.980948));
#14950=CARTESIAN_POINT('Ctrl Pts',(-0.0201990724523193,-0.246942143572133,
-0.980948));
#14951=CARTESIAN_POINT('Ctrl Pts',(-0.0421062857595697,-0.244251601209411,
-0.980270995488453));
#14952=CARTESIAN_POINT('Ctrl Pts',(-0.0842175114474171,-0.232861760990032,
-0.977553872336861));
#14953=CARTESIAN_POINT('Ctrl Pts',(-0.104422493053067,-0.224161999508995,
-0.975530745318961));
#14954=CARTESIAN_POINT('Ctrl Pts',(-0.139836317888042,-0.203463743702801,
-0.971100730005489));
#14955=CARTESIAN_POINT('Ctrl Pts',(-0.15681442133453,-0.190326085855194,
-0.968453058988463));
#14956=CARTESIAN_POINT('Ctrl Pts',(-0.1868781821531,-0.15976606450048,-0.963103647174702));
#14957=CARTESIAN_POINT('Ctrl Pts',(-0.199966927975188,-0.142345102874864,
-0.960411259488514));
#14958=CARTESIAN_POINT('Ctrl Pts',(-0.223801617934945,-0.099930567888331,
-0.955173119738174));
#14959=CARTESIAN_POINT('Ctrl Pts',(-0.233157223576062,-0.0740444353928835,
-0.952850216871763));
#14960=CARTESIAN_POINT('Ctrl Pts',(-0.238183666596899,-0.0476299999999999,
-0.951592097314));
#14961=CARTESIAN_POINT('Origin',(5.55111512312578E-17,-0.04763,-1.));
#14962=CARTESIAN_POINT('Origin',(0.,-0.04763,0.));
#14963=CARTESIAN_POINT('',(0.504455939115715,-0.04763,-0.841298510752802));
#14964=CARTESIAN_POINT('Origin',(0.,-0.04763,0.));
#14965=CARTESIAN_POINT('Origin',(0.707106781186548,-0.04763,-0.707106781186547));
#14966=CARTESIAN_POINT('Origin',(0.707106781186548,0.,-0.707106781186547));
#14967=CARTESIAN_POINT('',(0.841298510752802,-0.04763,-0.504455939115715));
#14968=CARTESIAN_POINT('Ctrl Pts',(0.841298510752802,-0.04763,-0.504455939115715));
#14969=CARTESIAN_POINT('Ctrl Pts',(0.838633903678357,-0.0740444353928835,
-0.508899795931835));
#14970=CARTESIAN_POINT('Ctrl Pts',(0.833661031856294,-0.0999305678883309,
-0.517157748491652));
#14971=CARTESIAN_POINT('Ctrl Pts',(0.820511285096538,-0.142345102874864,
-0.537715343527944));
#14972=CARTESIAN_POINT('Ctrl Pts',(0.813159949759,-0.159766064500479,-0.548874290046456));
#14973=CARTESIAN_POINT('Ctrl Pts',(0.795684265985088,-0.190326085855194,
-0.573915184558107));
#14974=CARTESIAN_POINT('Ctrl Pts',(0.78555112003688,-0.203463743702801,
-0.587792702767295));
#14975=CARTESIAN_POINT('Ctrl Pts',(0.763642258217233,-0.224161999508995,
-0.615966552324775));
#14976=CARTESIAN_POINT('Ctrl Pts',(0.750785745543687,-0.232861760990032,
-0.631684198665438));
#14977=CARTESIAN_POINT('Ctrl Pts',(0.722929908501543,-0.244251601209411,
-0.663382628119203));
#14978=CARTESIAN_POINT('Ctrl Pts',(0.707917883896095,-0.246942143572133,
-0.679352081686668));
#14979=CARTESIAN_POINT('Ctrl Pts',(0.679352081686668,-0.246942143572133,
-0.707917883896095));
#14980=CARTESIAN_POINT('Ctrl Pts',(0.663382628119203,-0.244251601209411,
-0.722929908501543));
#14981=CARTESIAN_POINT('Ctrl Pts',(0.631684198665438,-0.232861760990032,
-0.750785745543687));
#14982=CARTESIAN_POINT('Ctrl Pts',(0.615966552324775,-0.224161999508995,
-0.763642258217232));
#14983=CARTESIAN_POINT('Ctrl Pts',(0.587792702767295,-0.203463743702801,
-0.78555112003688));
#14984=CARTESIAN_POINT('Ctrl Pts',(0.573915184558107,-0.190326085855194,
-0.795684265985088));
#14985=CARTESIAN_POINT('Ctrl Pts',(0.548874290046456,-0.159766064500479,
-0.813159949759));
#14986=CARTESIAN_POINT('Ctrl Pts',(0.537715343527944,-0.142345102874864,
-0.820511285096538));
#14987=CARTESIAN_POINT('Ctrl Pts',(0.517157748491652,-0.099930567888331,
-0.833661031856294));
#14988=CARTESIAN_POINT('Ctrl Pts',(0.508899795931835,-0.0740444353928835,
-0.838633903678357));
#14989=CARTESIAN_POINT('Ctrl Pts',(0.504455939115715,-0.04763,-0.841298510752801));
#14990=CARTESIAN_POINT('Origin',(0.707106781186548,-0.04763,-0.707106781186547));
#14991=CARTESIAN_POINT('Origin',(0.,-0.166705,0.));
#14992=CARTESIAN_POINT('',(-0.980948,-0.28578,1.20131482833E-16));
#14993=CARTESIAN_POINT('Origin',(0.,-0.28578,0.));
#14994=CARTESIAN_POINT('',(-0.980948,-0.166705,1.20131482833E-16));
#14995=CARTESIAN_POINT('',(0.951592097314,-0.04763,0.238183666596899));
#14996=CARTESIAN_POINT('Origin',(0.,-0.04763,0.));
#14997=CARTESIAN_POINT('',(0.951592097314,-0.04763,-0.238183666596899));
#14998=CARTESIAN_POINT('Ctrl Pts',(0.951592097314,-0.04763,0.238183666596899));
#14999=CARTESIAN_POINT('Ctrl Pts',(0.952850216871763,-0.0740444353928835,
0.233157223576062));
#15000=CARTESIAN_POINT('Ctrl Pts',(0.955173119738174,-0.099930567888331,
0.223801617934945));
#15001=CARTESIAN_POINT('Ctrl Pts',(0.960411259488514,-0.142345102874864,
0.199966927975188));
#15002=CARTESIAN_POINT('Ctrl Pts',(0.963103647174702,-0.15976606450048,
0.1868781821531));
#15003=CARTESIAN_POINT('Ctrl Pts',(0.968453058988463,-0.190326085855194,
0.15681442133453));
#15004=CARTESIAN_POINT('Ctrl Pts',(0.971100730005489,-0.203463743702801,
0.139836317888042));
#15005=CARTESIAN_POINT('Ctrl Pts',(0.975530745318961,-0.224161999508995,
0.104422493053067));
#15006=CARTESIAN_POINT('Ctrl Pts',(0.977553872336861,-0.232861760990032,
0.0842175114474172));
#15007=CARTESIAN_POINT('Ctrl Pts',(0.980270995488453,-0.244251601209411,
0.0421062857595697));
#15008=CARTESIAN_POINT('Ctrl Pts',(0.980948,-0.246942143572133,0.0201990724523194));
#15009=CARTESIAN_POINT('Ctrl Pts',(0.980948,-0.246942143572133,-0.0201990724523194));
#15010=CARTESIAN_POINT('Ctrl Pts',(0.980270995488453,-0.244251601209411,
-0.0421062857595697));
#15011=CARTESIAN_POINT('Ctrl Pts',(0.977553872336861,-0.232861760990032,
-0.0842175114474172));
#15012=CARTESIAN_POINT('Ctrl Pts',(0.975530745318961,-0.224161999508995,
-0.104422493053067));
#15013=CARTESIAN_POINT('Ctrl Pts',(0.971100730005489,-0.203463743702801,
-0.139836317888042));
#15014=CARTESIAN_POINT('Ctrl Pts',(0.968453058988463,-0.190326085855194,
-0.15681442133453));
#15015=CARTESIAN_POINT('Ctrl Pts',(0.963103647174702,-0.15976606450048,
-0.1868781821531));
#15016=CARTESIAN_POINT('Ctrl Pts',(0.960411259488514,-0.142345102874864,
-0.199966927975188));
#15017=CARTESIAN_POINT('Ctrl Pts',(0.955173119738174,-0.099930567888331,
-0.223801617934945));
#15018=CARTESIAN_POINT('Ctrl Pts',(0.952850216871763,-0.0740444353928835,
-0.233157223576062));
#15019=CARTESIAN_POINT('Ctrl Pts',(0.951592097314,-0.0476299999999999,-0.238183666596899));
#15020=CARTESIAN_POINT('Origin',(0.,-0.04763,0.));
#15021=CARTESIAN_POINT('Origin',(0.,-0.04763,0.));
#15022=CARTESIAN_POINT('Origin',(1.,-0.04763,0.));
#15023=CARTESIAN_POINT('Origin',(1.,0.,0.));
#15024=CARTESIAN_POINT('Origin',(1.,-0.04763,0.));
#15025=CARTESIAN_POINT('Origin',(0.,-0.28578,0.));
#15026=CARTESIAN_POINT('Origin',(0.,-0.04763,0.));
#16567=UNCERTAINTY_MEASURE_WITH_UNIT(LENGTH_MEASURE(0.001),#16679,
'DISTANCE_ACCURACY_VALUE',
'Maximum model space distance between geometric entities at asserted c
onnectivities');
#16614=UNCERTAINTY_MEASURE_WITH_UNIT(LENGTH_MEASURE(0.001),#16679,
'DISTANCE_ACCURACY_VALUE',
'Maximum model space distance between geometric entities at asserted c
onnectivities');
#16631=(
GEOMETRIC_REPRESENTATION_CONTEXT(3)
GLOBAL_UNCERTAINTY_ASSIGNED_CONTEXT((#16567))
GLOBAL_UNIT_ASSIGNED_CONTEXT((#16679,#16681,#16682))
REPRESENTATION_CONTEXT('','3D')
);
#16678=(
GEOMETRIC_REPRESENTATION_CONTEXT(3)
GLOBAL_UNCERTAINTY_ASSIGNED_CONTEXT((#16614))
GLOBAL_UNIT_ASSIGNED_CONTEXT((#16679,#16681,#16682))
REPRESENTATION_CONTEXT('','3D')
);
#16679=(
LENGTH_UNIT()
NAMED_UNIT(*)
SI_UNIT(.CENTI.,.METRE.)
);
#16681=(
NAMED_UNIT(*)
PLANE_ANGLE_UNIT()
SI_UNIT($,.RADIAN.)
);
#16682=(
NAMED_UNIT(*)
SI_UNIT($,.STERADIAN.)
SOLID_ANGLE_UNIT()
);
#16699=SHAPE_DEFINITION_REPRESENTATION(#16762,#16926);
#16762=PRODUCT_DEFINITION_SHAPE('',$,#16990);
#16926=SHAPE_REPRESENTATION('',(#9846),#16631);
#16973=PRODUCT_DEFINITION_CONTEXT('part definition',#17164,'design');
#16990=PRODUCT_DEFINITION('Cage','Cage',#17053,#16973);
#17053=PRODUCT_DEFINITION_FORMATION('',$,#17182);
#17164=APPLICATION_CONTEXT(
'Core Data for Automotive Mechanical Design Process');
#17165=PRODUCT_CONTEXT('part definition',#17164,'mechanical');
#17182=PRODUCT('Cage','Cage','Cage',(#17165));
#17285=COLOUR_RGB('Grey',0.48,0.52,0.57);
#17286=FILL_AREA_STYLE_COLOUR('',#17285);
#17287=FILL_AREA_STYLE('',(#17286));
#17288=SURFACE_STYLE_FILL_AREA(#17287);
#17289=SURFACE_SIDE_STYLE('',(#17288));
#17290=SURFACE_STYLE_USAGE(.BOTH.,#17289);
#17291=PRESENTATION_STYLE_ASSIGNMENT((#17290));
ENDSEC;
END-ISO-10303-21;
